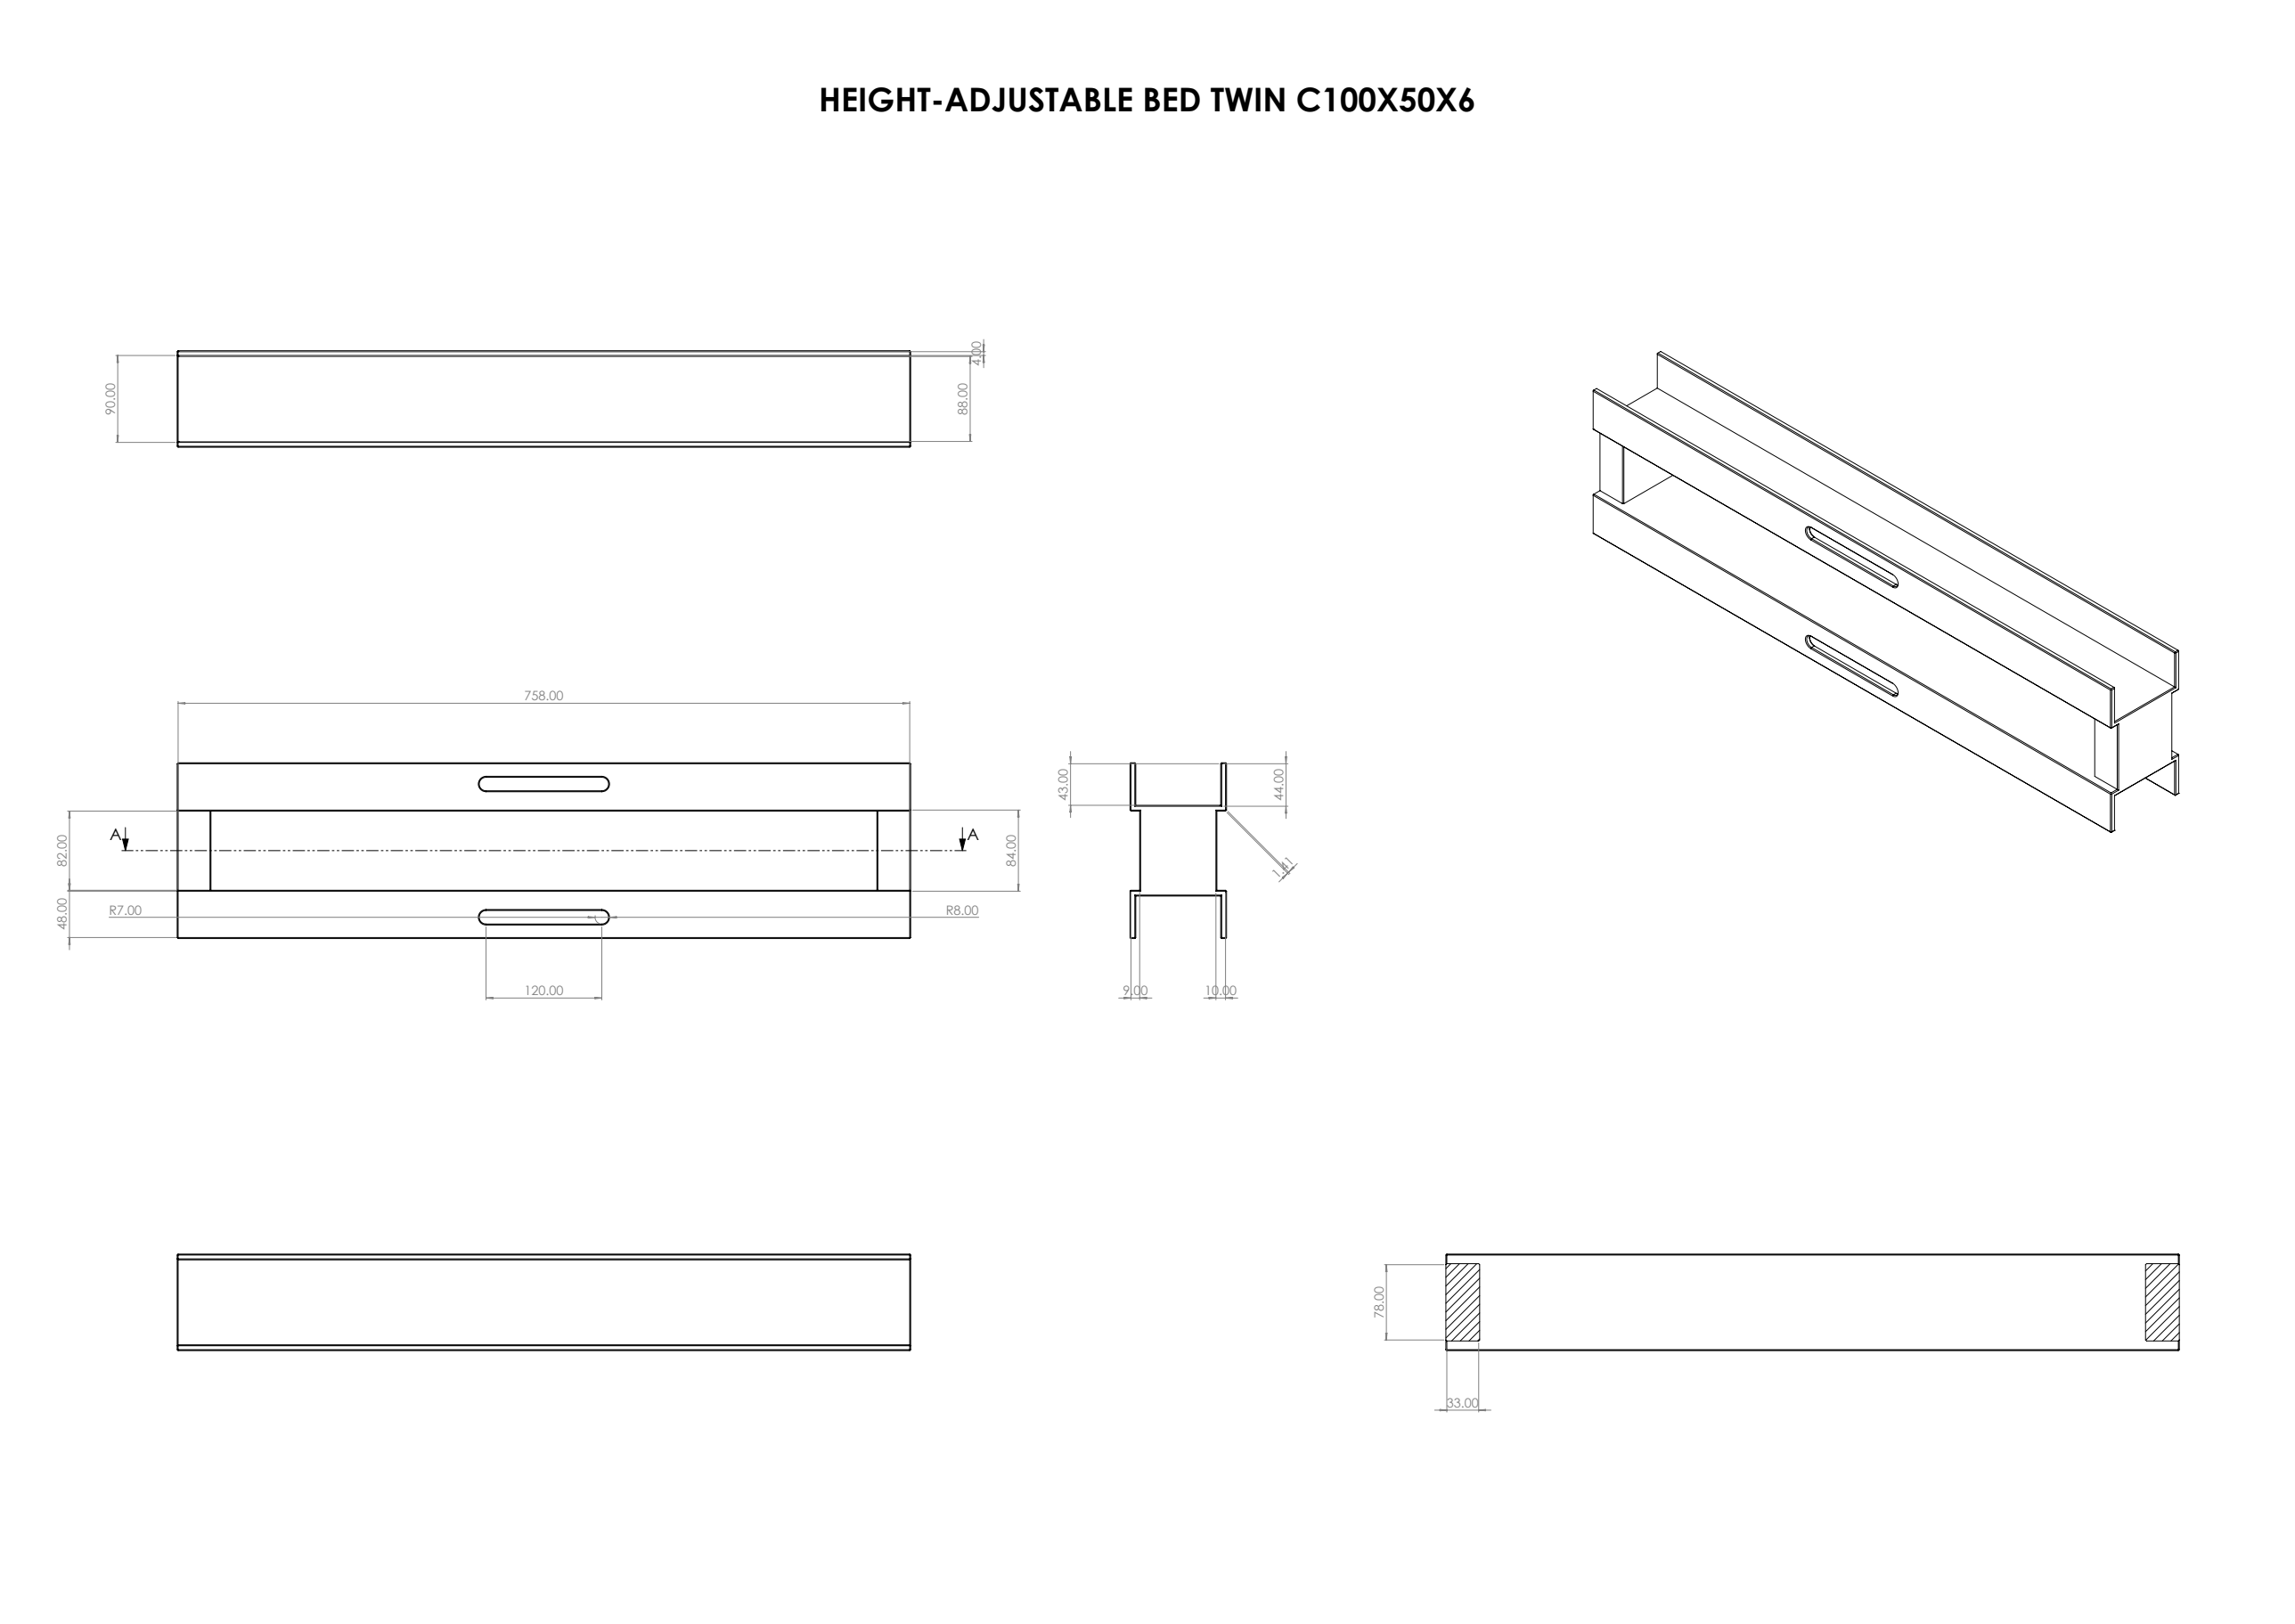
ISO-10303-21;
HEADER;
/* Generated by software containing ST-Developer
 * from STEP Tools, Inc. (www.steptools.com) 
 */

FILE_DESCRIPTION(
/* description */ (''),
/* implementation_level */ '2;1');

FILE_NAME(
/* name */ '04_Height-Adjustable_Bed_Twin_C100x50x6.step',
/* time_stamp */ '2026-10-20T10:03:03-07:00',
/* author */ (''),
/* organization */ (''),
/* preprocessor_version */ 'ST-DEVELOPER v20.2',
/* originating_system */ 'Autodesk Translation Framework v15.15.0.0',
/* authorisation */ '');

FILE_SCHEMA (('AUTOMOTIVE_DESIGN { 1 0 10303 214 3 1 1 }'));
ENDSEC;

DATA;
#10=MECHANICAL_DESIGN_GEOMETRIC_PRESENTATION_REPRESENTATION('',(#526),#71492);
#384=SHAPE_REPRESENTATION_RELATIONSHIP('SRR','None',#71605,#403);
#403=ADVANCED_BREP_SHAPE_REPRESENTATION('',(#422),#71475);
#422=MANIFOLD_SOLID_BREP('Bed',#28461);
#526=STYLED_ITEM('',(#71901),#422);
#1569=CYLINDRICAL_SURFACE('',#29276,0.7);
#1570=CYLINDRICAL_SURFACE('',#29284,0.699999999999999);
#1571=CYLINDRICAL_SURFACE('',#29291,0.699999999999999);
#1572=CYLINDRICAL_SURFACE('',#29299,0.7);
#1910=FACE_BOUND('',#5064,.T.);
#1911=FACE_BOUND('',#5070,.T.);
#1912=FACE_BOUND('',#5091,.T.);
#1913=FACE_BOUND('',#5097,.T.);
#2214=CIRCLE('',#29232,0.799999999999999);
#2215=CIRCLE('',#29233,0.8);
#2216=CIRCLE('',#29239,0.8);
#2217=CIRCLE('',#29240,0.799999999999999);
#2218=CIRCLE('',#29261,0.799999999999999);
#2219=CIRCLE('',#29262,0.8);
#2220=CIRCLE('',#29268,0.8);
#2221=CIRCLE('',#29269,0.799999999999999);
#2222=CIRCLE('',#29272,0.7);
#2223=CIRCLE('',#29275,0.699999999999999);
#2224=CIRCLE('',#29277,0.7);
#2225=CIRCLE('',#29281,0.699999999999999);
#2226=CIRCLE('',#29287,0.699999999999999);
#2227=CIRCLE('',#29290,0.7);
#2228=CIRCLE('',#29292,0.699999999999999);
#2229=CIRCLE('',#29296,0.7);
#2807=CONICAL_SURFACE('',#29271,0.75,0.785398163397475);
#2808=CONICAL_SURFACE('',#29274,0.749999999999999,0.785398163397475);
#2809=CONICAL_SURFACE('',#29280,0.749999999999999,0.785398163397475);
#2810=CONICAL_SURFACE('',#29283,0.75,0.785398163397475);
#2811=CONICAL_SURFACE('',#29286,0.749999999999999,0.785398163397475);
#2812=CONICAL_SURFACE('',#29289,0.75,0.785398163397475);
#2813=CONICAL_SURFACE('',#29295,0.75,0.785398163397475);
#2814=CONICAL_SURFACE('',#29298,0.749999999999999,0.785398163397475);
#3398=FACE_OUTER_BOUND('',#5014,.T.);
#3399=FACE_OUTER_BOUND('',#5015,.T.);
#3400=FACE_OUTER_BOUND('',#5016,.T.);
#3401=FACE_OUTER_BOUND('',#5017,.T.);
#3402=FACE_OUTER_BOUND('',#5018,.T.);
#3403=FACE_OUTER_BOUND('',#5019,.T.);
#3404=FACE_OUTER_BOUND('',#5020,.T.);
#3405=FACE_OUTER_BOUND('',#5021,.T.);
#3406=FACE_OUTER_BOUND('',#5022,.T.);
#3407=FACE_OUTER_BOUND('',#5023,.T.);
#3408=FACE_OUTER_BOUND('',#5024,.T.);
#3409=FACE_OUTER_BOUND('',#5025,.T.);
#3410=FACE_OUTER_BOUND('',#5026,.T.);
#3411=FACE_OUTER_BOUND('',#5027,.T.);
#3412=FACE_OUTER_BOUND('',#5028,.T.);
#3413=FACE_OUTER_BOUND('',#5029,.T.);
#3414=FACE_OUTER_BOUND('',#5030,.T.);
#3415=FACE_OUTER_BOUND('',#5031,.T.);
#3416=FACE_OUTER_BOUND('',#5032,.T.);
#3417=FACE_OUTER_BOUND('',#5033,.T.);
#3418=FACE_OUTER_BOUND('',#5034,.T.);
#3419=FACE_OUTER_BOUND('',#5035,.T.);
#3420=FACE_OUTER_BOUND('',#5036,.T.);
#3421=FACE_OUTER_BOUND('',#5037,.T.);
#3422=FACE_OUTER_BOUND('',#5038,.T.);
#3423=FACE_OUTER_BOUND('',#5039,.T.);
#3424=FACE_OUTER_BOUND('',#5040,.T.);
#3425=FACE_OUTER_BOUND('',#5041,.T.);
#3426=FACE_OUTER_BOUND('',#5042,.T.);
#3427=FACE_OUTER_BOUND('',#5043,.T.);
#3428=FACE_OUTER_BOUND('',#5044,.T.);
#3429=FACE_OUTER_BOUND('',#5045,.T.);
#3430=FACE_OUTER_BOUND('',#5046,.T.);
#3431=FACE_OUTER_BOUND('',#5047,.T.);
#3432=FACE_OUTER_BOUND('',#5048,.T.);
#3433=FACE_OUTER_BOUND('',#5049,.T.);
#3434=FACE_OUTER_BOUND('',#5050,.T.);
#3435=FACE_OUTER_BOUND('',#5051,.T.);
#3436=FACE_OUTER_BOUND('',#5052,.T.);
#3437=FACE_OUTER_BOUND('',#5053,.T.);
#3438=FACE_OUTER_BOUND('',#5054,.T.);
#3439=FACE_OUTER_BOUND('',#5055,.T.);
#3440=FACE_OUTER_BOUND('',#5056,.T.);
#3441=FACE_OUTER_BOUND('',#5057,.T.);
#3442=FACE_OUTER_BOUND('',#5058,.T.);
#3443=FACE_OUTER_BOUND('',#5059,.T.);
#3444=FACE_OUTER_BOUND('',#5060,.T.);
#3445=FACE_OUTER_BOUND('',#5061,.T.);
#3446=FACE_OUTER_BOUND('',#5062,.T.);
#3447=FACE_OUTER_BOUND('',#5063,.T.);
#3448=FACE_OUTER_BOUND('',#5065,.T.);
#3449=FACE_OUTER_BOUND('',#5066,.T.);
#3450=FACE_OUTER_BOUND('',#5067,.T.);
#3451=FACE_OUTER_BOUND('',#5068,.T.);
#3452=FACE_OUTER_BOUND('',#5069,.T.);
#3453=FACE_OUTER_BOUND('',#5071,.T.);
#3454=FACE_OUTER_BOUND('',#5072,.T.);
#3455=FACE_OUTER_BOUND('',#5073,.T.);
#3456=FACE_OUTER_BOUND('',#5074,.T.);
#3457=FACE_OUTER_BOUND('',#5075,.T.);
#3458=FACE_OUTER_BOUND('',#5076,.T.);
#3459=FACE_OUTER_BOUND('',#5077,.T.);
#3460=FACE_OUTER_BOUND('',#5078,.T.);
#3461=FACE_OUTER_BOUND('',#5079,.T.);
#3462=FACE_OUTER_BOUND('',#5080,.T.);
#3463=FACE_OUTER_BOUND('',#5081,.T.);
#3464=FACE_OUTER_BOUND('',#5082,.T.);
#3465=FACE_OUTER_BOUND('',#5083,.T.);
#3466=FACE_OUTER_BOUND('',#5084,.T.);
#3467=FACE_OUTER_BOUND('',#5085,.T.);
#3468=FACE_OUTER_BOUND('',#5086,.T.);
#3469=FACE_OUTER_BOUND('',#5087,.T.);
#3470=FACE_OUTER_BOUND('',#5088,.T.);
#3471=FACE_OUTER_BOUND('',#5089,.T.);
#3472=FACE_OUTER_BOUND('',#5090,.T.);
#3473=FACE_OUTER_BOUND('',#5092,.T.);
#3474=FACE_OUTER_BOUND('',#5093,.T.);
#3475=FACE_OUTER_BOUND('',#5094,.T.);
#3476=FACE_OUTER_BOUND('',#5095,.T.);
#3477=FACE_OUTER_BOUND('',#5096,.T.);
#3478=FACE_OUTER_BOUND('',#5098,.T.);
#3479=FACE_OUTER_BOUND('',#5099,.T.);
#3480=FACE_OUTER_BOUND('',#5100,.T.);
#3481=FACE_OUTER_BOUND('',#5101,.T.);
#3482=FACE_OUTER_BOUND('',#5102,.T.);
#3483=FACE_OUTER_BOUND('',#5103,.T.);
#3484=FACE_OUTER_BOUND('',#5104,.T.);
#3485=FACE_OUTER_BOUND('',#5105,.T.);
#3486=FACE_OUTER_BOUND('',#5106,.T.);
#3487=FACE_OUTER_BOUND('',#5107,.T.);
#3488=FACE_OUTER_BOUND('',#5108,.T.);
#3489=FACE_OUTER_BOUND('',#5109,.T.);
#3490=FACE_OUTER_BOUND('',#5110,.T.);
#3491=FACE_OUTER_BOUND('',#5111,.T.);
#3492=FACE_OUTER_BOUND('',#5112,.T.);
#3493=FACE_OUTER_BOUND('',#5113,.T.);
#3494=FACE_OUTER_BOUND('',#5114,.T.);
#3495=FACE_OUTER_BOUND('',#5115,.T.);
#3496=FACE_OUTER_BOUND('',#5116,.T.);
#3497=FACE_OUTER_BOUND('',#5117,.T.);
#3498=FACE_OUTER_BOUND('',#5118,.T.);
#3499=FACE_OUTER_BOUND('',#5119,.T.);
#3500=FACE_OUTER_BOUND('',#5120,.T.);
#3501=FACE_OUTER_BOUND('',#5121,.T.);
#3502=FACE_OUTER_BOUND('',#5122,.T.);
#3503=FACE_OUTER_BOUND('',#5123,.T.);
#3504=FACE_OUTER_BOUND('',#5124,.T.);
#3505=FACE_OUTER_BOUND('',#5125,.T.);
#5014=EDGE_LOOP('',(#20251,#20252,#20253,#20254));
#5015=EDGE_LOOP('',(#20255,#20256,#20257,#20258));
#5016=EDGE_LOOP('',(#20259,#20260,#20261,#20262,#20263,#20264));
#5017=EDGE_LOOP('',(#20265,#20266,#20267,#20268));
#5018=EDGE_LOOP('',(#20269,#20270,#20271,#20272,#20273,#20274));
#5019=EDGE_LOOP('',(#20275,#20276,#20277,#20278,#20279,#20280));
#5020=EDGE_LOOP('',(#20281,#20282,#20283,#20284));
#5021=EDGE_LOOP('',(#20285,#20286,#20287,#20288));
#5022=EDGE_LOOP('',(#20289,#20290,#20291,#20292));
#5023=EDGE_LOOP('',(#20293,#20294,#20295,#20296));
#5024=EDGE_LOOP('',(#20297,#20298,#20299,#20300,#20301,#20302));
#5025=EDGE_LOOP('',(#20303,#20304,#20305,#20306,#20307,#20308));
#5026=EDGE_LOOP('',(#20309,#20310,#20311,#20312));
#5027=EDGE_LOOP('',(#20313,#20314,#20315,#20316,#20317,#20318));
#5028=EDGE_LOOP('',(#20319,#20320,#20321,#20322,#20323,#20324));
#5029=EDGE_LOOP('',(#20325,#20326,#20327,#20328,#20329));
#5030=EDGE_LOOP('',(#20330,#20331,#20332,#20333));
#5031=EDGE_LOOP('',(#20334,#20335,#20336,#20337,#20338,#20339));
#5032=EDGE_LOOP('',(#20340,#20341,#20342,#20343,#20344));
#5033=EDGE_LOOP('',(#20345,#20346,#20347,#20348));
#5034=EDGE_LOOP('',(#20349,#20350,#20351,#20352));
#5035=EDGE_LOOP('',(#20353,#20354,#20355,#20356));
#5036=EDGE_LOOP('',(#20357,#20358,#20359,#20360));
#5037=EDGE_LOOP('',(#20361,#20362,#20363,#20364));
#5038=EDGE_LOOP('',(#20365,#20366,#20367));
#5039=EDGE_LOOP('',(#20368,#20369,#20370,#20371,#20372));
#5040=EDGE_LOOP('',(#20373,#20374,#20375));
#5041=EDGE_LOOP('',(#20376,#20377,#20378,#20379,#20380));
#5042=EDGE_LOOP('',(#20381,#20382,#20383,#20384,#20385));
#5043=EDGE_LOOP('',(#20386,#20387,#20388,#20389));
#5044=EDGE_LOOP('',(#20390,#20391,#20392,#20393));
#5045=EDGE_LOOP('',(#20394,#20395,#20396,#20397));
#5046=EDGE_LOOP('',(#20398,#20399,#20400,#20401,#20402));
#5047=EDGE_LOOP('',(#20403,#20404,#20405,#20406,#20407,#20408,#20409,#20410,
#20411,#20412,#20413,#20414,#20415,#20416,#20417,#20418,#20419,#20420,#20421,
#20422));
#5048=EDGE_LOOP('',(#20423,#20424,#20425,#20426,#20427,#20428));
#5049=EDGE_LOOP('',(#20429,#20430,#20431,#20432,#20433));
#5050=EDGE_LOOP('',(#20434,#20435,#20436,#20437));
#5051=EDGE_LOOP('',(#20438,#20439,#20440,#20441,#20442));
#5052=EDGE_LOOP('',(#20443,#20444,#20445,#20446));
#5053=EDGE_LOOP('',(#20447,#20448,#20449,#20450,#20451));
#5054=EDGE_LOOP('',(#20452,#20453,#20454,#20455));
#5055=EDGE_LOOP('',(#20456,#20457,#20458));
#5056=EDGE_LOOP('',(#20459,#20460,#20461,#20462,#20463));
#5057=EDGE_LOOP('',(#20464,#20465,#20466,#20467));
#5058=EDGE_LOOP('',(#20468,#20469,#20470,#20471,#20472));
#5059=EDGE_LOOP('',(#20473,#20474,#20475,#20476));
#5060=EDGE_LOOP('',(#20477,#20478,#20479,#20480,#20481,#20482,#20483,#20484,
#20485,#20486,#20487,#20488,#20489,#20490,#20491,#20492));
#5061=EDGE_LOOP('',(#20493,#20494,#20495,#20496,#20497));
#5062=EDGE_LOOP('',(#20498,#20499,#20500,#20501,#20502,#20503));
#5063=EDGE_LOOP('',(#20504,#20505,#20506,#20507));
#5064=EDGE_LOOP('',(#20508,#20509,#20510,#20511));
#5065=EDGE_LOOP('',(#20512,#20513,#20514,#20515,#20516,#20517));
#5066=EDGE_LOOP('',(#20518,#20519,#20520,#20521,#20522,#20523));
#5067=EDGE_LOOP('',(#20524,#20525,#20526,#20527,#20528,#20529));
#5068=EDGE_LOOP('',(#20530,#20531,#20532,#20533,#20534));
#5069=EDGE_LOOP('',(#20535,#20536,#20537,#20538));
#5070=EDGE_LOOP('',(#20539,#20540,#20541,#20542));
#5071=EDGE_LOOP('',(#20543,#20544,#20545,#20546,#20547));
#5072=EDGE_LOOP('',(#20548,#20549,#20550,#20551,#20552,#20553));
#5073=EDGE_LOOP('',(#20554,#20555,#20556,#20557));
#5074=EDGE_LOOP('',(#20558,#20559,#20560,#20561,#20562));
#5075=EDGE_LOOP('',(#20563,#20564,#20565,#20566,#20567,#20568,#20569,#20570,
#20571,#20572,#20573,#20574,#20575,#20576,#20577,#20578,#20579,#20580,#20581,
#20582));
#5076=EDGE_LOOP('',(#20583,#20584,#20585,#20586));
#5077=EDGE_LOOP('',(#20587,#20588,#20589,#20590));
#5078=EDGE_LOOP('',(#20591,#20592,#20593));
#5079=EDGE_LOOP('',(#20594,#20595,#20596,#20597));
#5080=EDGE_LOOP('',(#20598,#20599,#20600,#20601,#20602));
#5081=EDGE_LOOP('',(#20603,#20604,#20605,#20606,#20607));
#5082=EDGE_LOOP('',(#20608,#20609,#20610,#20611));
#5083=EDGE_LOOP('',(#20612,#20613,#20614,#20615,#20616,#20617));
#5084=EDGE_LOOP('',(#20618,#20619,#20620,#20621));
#5085=EDGE_LOOP('',(#20622,#20623,#20624,#20625,#20626,#20627,#20628,#20629,
#20630,#20631,#20632,#20633,#20634,#20635,#20636,#20637));
#5086=EDGE_LOOP('',(#20638,#20639,#20640,#20641,#20642,#20643));
#5087=EDGE_LOOP('',(#20644,#20645,#20646,#20647));
#5088=EDGE_LOOP('',(#20648,#20649,#20650,#20651,#20652));
#5089=EDGE_LOOP('',(#20653,#20654,#20655,#20656,#20657));
#5090=EDGE_LOOP('',(#20658,#20659,#20660,#20661));
#5091=EDGE_LOOP('',(#20662,#20663,#20664,#20665));
#5092=EDGE_LOOP('',(#20666,#20667,#20668,#20669,#20670,#20671));
#5093=EDGE_LOOP('',(#20672,#20673,#20674,#20675,#20676));
#5094=EDGE_LOOP('',(#20677,#20678,#20679,#20680,#20681,#20682));
#5095=EDGE_LOOP('',(#20683,#20684,#20685,#20686,#20687,#20688));
#5096=EDGE_LOOP('',(#20689,#20690,#20691,#20692));
#5097=EDGE_LOOP('',(#20693,#20694,#20695,#20696));
#5098=EDGE_LOOP('',(#20697,#20698,#20699,#20700));
#5099=EDGE_LOOP('',(#20701,#20702,#20703,#20704));
#5100=EDGE_LOOP('',(#20705,#20706,#20707,#20708));
#5101=EDGE_LOOP('',(#20709,#20710,#20711,#20712));
#5102=EDGE_LOOP('',(#20713,#20714,#20715,#20716));
#5103=EDGE_LOOP('',(#20717,#20718,#20719,#20720));
#5104=EDGE_LOOP('',(#20721,#20722,#20723,#20724));
#5105=EDGE_LOOP('',(#20725,#20726,#20727,#20728));
#5106=EDGE_LOOP('',(#20729,#20730,#20731,#20732));
#5107=EDGE_LOOP('',(#20733,#20734,#20735,#20736));
#5108=EDGE_LOOP('',(#20737,#20738,#20739,#20740));
#5109=EDGE_LOOP('',(#20741,#20742,#20743,#20744));
#5110=EDGE_LOOP('',(#20745,#20746,#20747,#20748));
#5111=EDGE_LOOP('',(#20749,#20750,#20751,#20752));
#5112=EDGE_LOOP('',(#20753,#20754,#20755,#20756));
#5113=EDGE_LOOP('',(#20757,#20758,#20759,#20760));
#5114=EDGE_LOOP('',(#20761,#20762,#20763,#20764));
#5115=EDGE_LOOP('',(#20765,#20766,#20767,#20768));
#5116=EDGE_LOOP('',(#20769,#20770,#20771,#20772));
#5117=EDGE_LOOP('',(#20773,#20774,#20775,#20776));
#5118=EDGE_LOOP('',(#20777,#20778,#20779,#20780));
#5119=EDGE_LOOP('',(#20781,#20782,#20783,#20784));
#5120=EDGE_LOOP('',(#20785,#20786,#20787,#20788));
#5121=EDGE_LOOP('',(#20789,#20790,#20791,#20792));
#5122=EDGE_LOOP('',(#20793,#20794,#20795,#20796));
#5123=EDGE_LOOP('',(#20797,#20798,#20799,#20800,#20801,#20802));
#5124=EDGE_LOOP('',(#20803,#20804,#20805,#20806));
#5125=EDGE_LOOP('',(#20807,#20808,#20809,#20810));
#7065=LINE('',#42807,#9553);
#7066=LINE('',#42809,#9554);
#7067=LINE('',#42811,#9555);
#7068=LINE('',#42812,#9556);
#7069=LINE('',#42815,#9557);
#7070=LINE('',#42817,#9558);
#7071=LINE('',#42818,#9559);
#7072=LINE('',#42822,#9560);
#7073=LINE('',#42824,#9561);
#7074=LINE('',#42826,#9562);
#7075=LINE('',#42828,#9563);
#7076=LINE('',#42830,#9564);
#7077=LINE('',#42831,#9565);
#7078=LINE('',#42834,#9566);
#7079=LINE('',#42836,#9567);
#7080=LINE('',#42837,#9568);
#7081=LINE('',#42840,#9569);
#7082=LINE('',#42842,#9570);
#7083=LINE('',#42844,#9571);
#7084=LINE('',#42845,#9572);
#7085=LINE('',#42848,#9573);
#7086=LINE('',#42850,#9574);
#7087=LINE('',#42852,#9575);
#7088=LINE('',#42853,#9576);
#7089=LINE('',#42857,#9577);
#7090=LINE('',#42859,#9578);
#7091=LINE('',#42861,#9579);
#7092=LINE('',#42862,#9580);
#7093=LINE('',#42864,#9581);
#7094=LINE('',#42865,#9582);
#7095=LINE('',#42869,#9583);
#7096=LINE('',#42871,#9584);
#7097=LINE('',#42873,#9585);
#7098=LINE('',#42874,#9586);
#7099=LINE('',#42877,#9587);
#7100=LINE('',#42879,#9588);
#7101=LINE('',#42880,#9589);
#7102=LINE('',#42884,#9590);
#7103=LINE('',#42886,#9591);
#7104=LINE('',#42888,#9592);
#7105=LINE('',#42890,#9593);
#7106=LINE('',#42892,#9594);
#7107=LINE('',#42893,#9595);
#7108=LINE('',#42896,#9596);
#7109=LINE('',#42898,#9597);
#7110=LINE('',#42900,#9598);
#7111=LINE('',#42902,#9599);
#7112=LINE('',#42903,#9600);
#7113=LINE('',#42906,#9601);
#7114=LINE('',#42907,#9602);
#7115=LINE('',#42910,#9603);
#7116=LINE('',#42912,#9604);
#7117=LINE('',#42914,#9605);
#7118=LINE('',#42915,#9606);
#7119=LINE('',#42918,#9607);
#7120=LINE('',#42920,#9608);
#7121=LINE('',#42921,#9609);
#7122=LINE('',#42924,#9610);
#7123=LINE('',#42926,#9611);
#7124=LINE('',#42927,#9612);
#7125=LINE('',#42930,#9613);
#7126=LINE('',#42931,#9614);
#7127=LINE('',#42934,#9615);
#7128=LINE('',#42936,#9616);
#7129=LINE('',#42937,#9617);
#7130=LINE('',#42940,#9618);
#7131=LINE('',#42942,#9619);
#7132=LINE('',#42943,#9620);
#7133=LINE('',#42946,#9621);
#7134=LINE('',#42948,#9622);
#7135=LINE('',#42949,#9623);
#7136=LINE('',#42952,#9624);
#7137=LINE('',#42953,#9625);
#7138=LINE('',#42956,#9626);
#7139=LINE('',#42957,#9627);
#7140=LINE('',#42961,#9628);
#7141=LINE('',#42963,#9629);
#7142=LINE('',#42965,#9630);
#7143=LINE('',#42966,#9631);
#7144=LINE('',#42968,#9632);
#7145=LINE('',#42969,#9633);
#7146=LINE('',#42972,#9634);
#7147=LINE('',#42973,#9635);
#7148=LINE('',#42976,#9636);
#7149=LINE('',#42977,#9637);
#7150=LINE('',#42981,#9638);
#7151=LINE('',#42983,#9639);
#7152=LINE('',#42984,#9640);
#7153=LINE('',#42986,#9641);
#7154=LINE('',#42988,#9642);
#7155=LINE('',#42989,#9643);
#7156=LINE('',#42992,#9644);
#7157=LINE('',#42993,#9645);
#7158=LINE('',#42994,#9646);
#7159=LINE('',#42996,#9647);
#7160=LINE('',#42998,#9648);
#7161=LINE('',#42999,#9649);
#7162=LINE('',#43002,#9650);
#7163=LINE('',#43003,#9651);
#7164=LINE('',#43005,#9652);
#7165=LINE('',#43006,#9653);
#7166=LINE('',#43009,#9654);
#7167=LINE('',#43010,#9655);
#7168=LINE('',#43011,#9656);
#7169=LINE('',#43014,#9657);
#7170=LINE('',#43016,#9658);
#7171=LINE('',#43018,#9659);
#7172=LINE('',#43020,#9660);
#7173=LINE('',#43022,#9661);
#7174=LINE('',#43024,#9662);
#7175=LINE('',#43026,#9663);
#7176=LINE('',#43028,#9664);
#7177=LINE('',#43030,#9665);
#7178=LINE('',#43032,#9666);
#7179=LINE('',#43034,#9667);
#7180=LINE('',#43035,#9668);
#7181=LINE('',#43038,#9669);
#7182=LINE('',#43040,#9670);
#7183=LINE('',#43042,#9671);
#7184=LINE('',#43043,#9672);
#7185=LINE('',#43046,#9673);
#7186=LINE('',#43047,#9674);
#7187=LINE('',#43048,#9675);
#7188=LINE('',#43051,#9676);
#7189=LINE('',#43052,#9677);
#7190=LINE('',#43055,#9678);
#7191=LINE('',#43056,#9679);
#7192=LINE('',#43059,#9680);
#7193=LINE('',#43060,#9681);
#7194=LINE('',#43064,#9682);
#7195=LINE('',#43066,#9683);
#7196=LINE('',#43067,#9684);
#7197=LINE('',#43068,#9685);
#7198=LINE('',#43071,#9686);
#7199=LINE('',#43072,#9687);
#7200=LINE('',#43075,#9688);
#7201=LINE('',#43077,#9689);
#7202=LINE('',#43078,#9690);
#7203=LINE('',#43082,#9691);
#7204=LINE('',#43083,#9692);
#7205=LINE('',#43085,#9693);
#7206=LINE('',#43086,#9694);
#7207=LINE('',#43088,#9695);
#7208=LINE('',#43092,#9696);
#7209=LINE('',#43093,#9697);
#7210=LINE('',#43094,#9698);
#7211=LINE('',#43096,#9699);
#7212=LINE('',#43097,#9700);
#7213=LINE('',#43100,#9701);
#7214=LINE('',#43101,#9702);
#7215=LINE('',#43102,#9703);
#7216=LINE('',#43105,#9704);
#7217=LINE('',#43107,#9705);
#7218=LINE('',#43108,#9706);
#7219=LINE('',#43111,#9707);
#7220=LINE('',#43113,#9708);
#7221=LINE('',#43115,#9709);
#7222=LINE('',#43116,#9710);
#7223=LINE('',#43118,#9711);
#7224=LINE('',#43121,#9712);
#7225=LINE('',#43125,#9713);
#7226=LINE('',#43129,#9714);
#7227=LINE('',#43131,#9715);
#7228=LINE('',#43132,#9716);
#7229=LINE('',#43135,#9717);
#7230=LINE('',#43137,#9718);
#7231=LINE('',#43139,#9719);
#7232=LINE('',#43140,#9720);
#7233=LINE('',#43144,#9721);
#7234=LINE('',#43146,#9722);
#7235=LINE('',#43147,#9723);
#7236=LINE('',#43149,#9724);
#7237=LINE('',#43150,#9725);
#7238=LINE('',#43153,#9726);
#7239=LINE('',#43155,#9727);
#7240=LINE('',#43156,#9728);
#7241=LINE('',#43158,#9729);
#7242=LINE('',#43159,#9730);
#7243=LINE('',#43162,#9731);
#7244=LINE('',#43166,#9732);
#7245=LINE('',#43169,#9733);
#7246=LINE('',#43171,#9734);
#7247=LINE('',#43174,#9735);
#7248=LINE('',#43175,#9736);
#7249=LINE('',#43177,#9737);
#7250=LINE('',#43180,#9738);
#7251=LINE('',#43182,#9739);
#7252=LINE('',#43184,#9740);
#7253=LINE('',#43186,#9741);
#7254=LINE('',#43188,#9742);
#7255=LINE('',#43190,#9743);
#7256=LINE('',#43191,#9744);
#7257=LINE('',#43192,#9745);
#7258=LINE('',#43194,#9746);
#7259=LINE('',#43199,#9747);
#7260=LINE('',#43200,#9748);
#7261=LINE('',#43201,#9749);
#7262=LINE('',#43204,#9750);
#7263=LINE('',#43205,#9751);
#7264=LINE('',#43209,#9752);
#7265=LINE('',#43210,#9753);
#7266=LINE('',#43211,#9754);
#7267=LINE('',#43213,#9755);
#7268=LINE('',#43215,#9756);
#7269=LINE('',#43216,#9757);
#7270=LINE('',#43218,#9758);
#7271=LINE('',#43221,#9759);
#7272=LINE('',#43223,#9760);
#7273=LINE('',#43224,#9761);
#7274=LINE('',#43226,#9762);
#7275=LINE('',#43230,#9763);
#7276=LINE('',#43232,#9764);
#7277=LINE('',#43234,#9765);
#7278=LINE('',#43235,#9766);
#7279=LINE('',#43237,#9767);
#7280=LINE('',#43238,#9768);
#7281=LINE('',#43242,#9769);
#7282=LINE('',#43243,#9770);
#7283=LINE('',#43246,#9771);
#7284=LINE('',#43247,#9772);
#7285=LINE('',#43250,#9773);
#7286=LINE('',#43254,#9774);
#7287=LINE('',#43258,#9775);
#7288=LINE('',#43260,#9776);
#7289=LINE('',#43261,#9777);
#7290=LINE('',#43263,#9778);
#7291=LINE('',#43266,#9779);
#7292=LINE('',#43267,#9780);
#7293=LINE('',#43269,#9781);
#7294=LINE('',#43270,#9782);
#7295=LINE('',#43274,#9783);
#7296=LINE('',#43278,#9784);
#7297=LINE('',#43282,#9785);
#7298=LINE('',#43284,#9786);
#7299=LINE('',#43285,#9787);
#7300=LINE('',#43288,#9788);
#7301=LINE('',#43292,#9789);
#7302=LINE('',#43293,#9790);
#7303=LINE('',#43298,#9791);
#7304=LINE('',#43301,#9792);
#7305=LINE('',#43304,#9793);
#7306=LINE('',#43305,#9794);
#7307=LINE('',#43307,#9795);
#7308=LINE('',#43308,#9796);
#7309=LINE('',#43311,#9797);
#7310=LINE('',#43314,#9798);
#7311=LINE('',#43315,#9799);
#7312=LINE('',#43318,#9800);
#7313=LINE('',#43321,#9801);
#7314=LINE('',#43323,#9802);
#7315=LINE('',#43324,#9803);
#7316=LINE('',#43327,#9804);
#7317=LINE('',#43331,#9805);
#7318=LINE('',#43332,#9806);
#7319=LINE('',#43337,#9807);
#7320=LINE('',#43340,#9808);
#7321=LINE('',#43343,#9809);
#7322=LINE('',#43344,#9810);
#7323=LINE('',#43346,#9811);
#7324=LINE('',#43347,#9812);
#7325=LINE('',#43350,#9813);
#7326=LINE('',#43353,#9814);
#7327=LINE('',#43354,#9815);
#7328=LINE('',#43357,#9816);
#9553=VECTOR('',#32608,1.);
#9554=VECTOR('',#32609,1.);
#9555=VECTOR('',#32610,1.);
#9556=VECTOR('',#32611,1.);
#9557=VECTOR('',#32614,1.);
#9558=VECTOR('',#32615,1.);
#9559=VECTOR('',#32616,1.);
#9560=VECTOR('',#32619,1.);
#9561=VECTOR('',#32620,1.);
#9562=VECTOR('',#32621,1.);
#9563=VECTOR('',#32622,1.);
#9564=VECTOR('',#32623,1.);
#9565=VECTOR('',#32624,1.);
#9566=VECTOR('',#32627,1.);
#9567=VECTOR('',#32628,1.);
#9568=VECTOR('',#32629,1.);
#9569=VECTOR('',#32632,1.);
#9570=VECTOR('',#32633,1.);
#9571=VECTOR('',#32634,1.);
#9572=VECTOR('',#32635,1.);
#9573=VECTOR('',#32638,1.);
#9574=VECTOR('',#32639,1.);
#9575=VECTOR('',#32640,1.);
#9576=VECTOR('',#32641,1.);
#9577=VECTOR('',#32644,1.);
#9578=VECTOR('',#32645,1.);
#9579=VECTOR('',#32646,1.);
#9580=VECTOR('',#32647,1.);
#9581=VECTOR('',#32650,1.);
#9582=VECTOR('',#32651,1.);
#9583=VECTOR('',#32654,1.);
#9584=VECTOR('',#32655,1.);
#9585=VECTOR('',#32656,1.);
#9586=VECTOR('',#32657,1.);
#9587=VECTOR('',#32660,1.);
#9588=VECTOR('',#32661,1.);
#9589=VECTOR('',#32662,1.);
#9590=VECTOR('',#32665,1.);
#9591=VECTOR('',#32666,1.);
#9592=VECTOR('',#32667,1.);
#9593=VECTOR('',#32668,1.);
#9594=VECTOR('',#32669,1.);
#9595=VECTOR('',#32670,1.);
#9596=VECTOR('',#32673,1.);
#9597=VECTOR('',#32674,1.);
#9598=VECTOR('',#32675,1.);
#9599=VECTOR('',#32676,1.);
#9600=VECTOR('',#32677,1.);
#9601=VECTOR('',#32680,1.);
#9602=VECTOR('',#32681,1.);
#9603=VECTOR('',#32684,1.);
#9604=VECTOR('',#32685,1.);
#9605=VECTOR('',#32686,1.);
#9606=VECTOR('',#32687,1.);
#9607=VECTOR('',#32690,1.);
#9608=VECTOR('',#32691,1.);
#9609=VECTOR('',#32692,1.);
#9610=VECTOR('',#32695,1.);
#9611=VECTOR('',#32696,1.);
#9612=VECTOR('',#32697,1.);
#9613=VECTOR('',#32700,1.);
#9614=VECTOR('',#32701,1.);
#9615=VECTOR('',#32704,1.);
#9616=VECTOR('',#32705,1.);
#9617=VECTOR('',#32706,1.);
#9618=VECTOR('',#32709,1.);
#9619=VECTOR('',#32710,1.);
#9620=VECTOR('',#32711,1.);
#9621=VECTOR('',#32714,1.);
#9622=VECTOR('',#32715,1.);
#9623=VECTOR('',#32716,1.);
#9624=VECTOR('',#32719,1.);
#9625=VECTOR('',#32720,1.);
#9626=VECTOR('',#32723,1.);
#9627=VECTOR('',#32724,1.);
#9628=VECTOR('',#32727,1.);
#9629=VECTOR('',#32728,1.);
#9630=VECTOR('',#32729,1.);
#9631=VECTOR('',#32730,1.);
#9632=VECTOR('',#32733,1.);
#9633=VECTOR('',#32734,1.);
#9634=VECTOR('',#32737,1.);
#9635=VECTOR('',#32738,1.);
#9636=VECTOR('',#32741,1.);
#9637=VECTOR('',#32742,1.);
#9638=VECTOR('',#32745,1.);
#9639=VECTOR('',#32746,1.);
#9640=VECTOR('',#32747,1.);
#9641=VECTOR('',#32750,1.);
#9642=VECTOR('',#32751,1.);
#9643=VECTOR('',#32752,1.);
#9644=VECTOR('',#32755,1.);
#9645=VECTOR('',#32756,1.);
#9646=VECTOR('',#32757,1.);
#9647=VECTOR('',#32760,1.);
#9648=VECTOR('',#32761,1.);
#9649=VECTOR('',#32762,1.);
#9650=VECTOR('',#32765,1.);
#9651=VECTOR('',#32766,1.);
#9652=VECTOR('',#32769,1.);
#9653=VECTOR('',#32770,1.);
#9654=VECTOR('',#32773,1.);
#9655=VECTOR('',#32774,1.);
#9656=VECTOR('',#32775,1.);
#9657=VECTOR('',#32778,1.);
#9658=VECTOR('',#32779,1.);
#9659=VECTOR('',#32780,1.);
#9660=VECTOR('',#32781,1.);
#9661=VECTOR('',#32782,1.);
#9662=VECTOR('',#32783,1.);
#9663=VECTOR('',#32784,1.);
#9664=VECTOR('',#32785,1.);
#9665=VECTOR('',#32786,1.);
#9666=VECTOR('',#32787,1.);
#9667=VECTOR('',#32788,1.);
#9668=VECTOR('',#32789,1.);
#9669=VECTOR('',#32792,1.);
#9670=VECTOR('',#32793,1.);
#9671=VECTOR('',#32794,1.);
#9672=VECTOR('',#32795,1.);
#9673=VECTOR('',#32798,1.);
#9674=VECTOR('',#32799,1.);
#9675=VECTOR('',#32800,1.);
#9676=VECTOR('',#32803,1.);
#9677=VECTOR('',#32804,1.);
#9678=VECTOR('',#32807,1.);
#9679=VECTOR('',#32808,1.);
#9680=VECTOR('',#32811,1.);
#9681=VECTOR('',#32812,1.);
#9682=VECTOR('',#32815,1.);
#9683=VECTOR('',#32816,1.);
#9684=VECTOR('',#32817,1.);
#9685=VECTOR('',#32818,1.);
#9686=VECTOR('',#32821,1.);
#9687=VECTOR('',#32822,1.);
#9688=VECTOR('',#32825,1.);
#9689=VECTOR('',#32826,1.);
#9690=VECTOR('',#32827,1.);
#9691=VECTOR('',#32830,1.);
#9692=VECTOR('',#32831,1.);
#9693=VECTOR('',#32832,1.);
#9694=VECTOR('',#32833,1.);
#9695=VECTOR('',#32836,1.);
#9696=VECTOR('',#32839,1.);
#9697=VECTOR('',#32840,1.);
#9698=VECTOR('',#32841,1.);
#9699=VECTOR('',#32844,1.);
#9700=VECTOR('',#32845,1.);
#9701=VECTOR('',#32848,1.);
#9702=VECTOR('',#32849,1.);
#9703=VECTOR('',#32850,1.);
#9704=VECTOR('',#32853,1.);
#9705=VECTOR('',#32854,1.);
#9706=VECTOR('',#32855,1.);
#9707=VECTOR('',#32858,1.);
#9708=VECTOR('',#32859,1.);
#9709=VECTOR('',#32860,1.);
#9710=VECTOR('',#32861,1.);
#9711=VECTOR('',#32864,1.);
#9712=VECTOR('',#32865,1.);
#9713=VECTOR('',#32868,1.);
#9714=VECTOR('',#32873,1.);
#9715=VECTOR('',#32874,1.);
#9716=VECTOR('',#32875,1.);
#9717=VECTOR('',#32878,1.);
#9718=VECTOR('',#32879,1.);
#9719=VECTOR('',#32880,1.);
#9720=VECTOR('',#32881,1.);
#9721=VECTOR('',#32884,1.);
#9722=VECTOR('',#32885,1.);
#9723=VECTOR('',#32886,1.);
#9724=VECTOR('',#32887,1.);
#9725=VECTOR('',#32888,1.);
#9726=VECTOR('',#32891,1.);
#9727=VECTOR('',#32892,1.);
#9728=VECTOR('',#32893,1.);
#9729=VECTOR('',#32896,1.);
#9730=VECTOR('',#32897,1.);
#9731=VECTOR('',#32898,1.);
#9732=VECTOR('',#32901,1.);
#9733=VECTOR('',#32906,1.);
#9734=VECTOR('',#32909,1.);
#9735=VECTOR('',#32912,1.);
#9736=VECTOR('',#32913,1.);
#9737=VECTOR('',#32916,1.);
#9738=VECTOR('',#32919,1.);
#9739=VECTOR('',#32920,1.);
#9740=VECTOR('',#32921,1.);
#9741=VECTOR('',#32922,1.);
#9742=VECTOR('',#32923,1.);
#9743=VECTOR('',#32924,1.);
#9744=VECTOR('',#32925,1.);
#9745=VECTOR('',#32926,1.);
#9746=VECTOR('',#32929,1.);
#9747=VECTOR('',#32934,1.);
#9748=VECTOR('',#32935,1.);
#9749=VECTOR('',#32936,1.);
#9750=VECTOR('',#32939,1.);
#9751=VECTOR('',#32940,1.);
#9752=VECTOR('',#32943,1.);
#9753=VECTOR('',#32944,1.);
#9754=VECTOR('',#32945,1.);
#9755=VECTOR('',#32948,1.);
#9756=VECTOR('',#32949,1.);
#9757=VECTOR('',#32950,1.);
#9758=VECTOR('',#32953,1.);
#9759=VECTOR('',#32956,1.);
#9760=VECTOR('',#32957,1.);
#9761=VECTOR('',#32958,1.);
#9762=VECTOR('',#32961,1.);
#9763=VECTOR('',#32966,1.);
#9764=VECTOR('',#32967,1.);
#9765=VECTOR('',#32968,1.);
#9766=VECTOR('',#32969,1.);
#9767=VECTOR('',#32972,1.);
#9768=VECTOR('',#32973,1.);
#9769=VECTOR('',#32978,1.);
#9770=VECTOR('',#32979,1.);
#9771=VECTOR('',#32982,1.);
#9772=VECTOR('',#32983,1.);
#9773=VECTOR('',#32984,1.);
#9774=VECTOR('',#32987,1.);
#9775=VECTOR('',#32992,1.);
#9776=VECTOR('',#32993,1.);
#9777=VECTOR('',#32994,1.);
#9778=VECTOR('',#32997,1.);
#9779=VECTOR('',#33000,1.);
#9780=VECTOR('',#33001,1.);
#9781=VECTOR('',#33004,1.);
#9782=VECTOR('',#33005,1.);
#9783=VECTOR('',#33008,1.);
#9784=VECTOR('',#33011,1.);
#9785=VECTOR('',#33016,1.);
#9786=VECTOR('',#33017,1.);
#9787=VECTOR('',#33018,1.);
#9788=VECTOR('',#33021,1.);
#9789=VECTOR('',#33026,1.);
#9790=VECTOR('',#33027,1.);
#9791=VECTOR('',#33034,1.);
#9792=VECTOR('',#33037,1.);
#9793=VECTOR('',#33040,1.);
#9794=VECTOR('',#33041,1.);
#9795=VECTOR('',#33044,1.);
#9796=VECTOR('',#33045,1.);
#9797=VECTOR('',#33048,1.);
#9798=VECTOR('',#33053,1.);
#9799=VECTOR('',#33054,1.);
#9800=VECTOR('',#33059,1.);
#9801=VECTOR('',#33062,1.);
#9802=VECTOR('',#33063,1.);
#9803=VECTOR('',#33064,1.);
#9804=VECTOR('',#33067,1.);
#9805=VECTOR('',#33072,1.);
#9806=VECTOR('',#33073,1.);
#9807=VECTOR('',#33080,1.);
#9808=VECTOR('',#33083,1.);
#9809=VECTOR('',#33086,1.);
#9810=VECTOR('',#33087,1.);
#9811=VECTOR('',#33090,1.);
#9812=VECTOR('',#33091,1.);
#9813=VECTOR('',#33094,1.);
#9814=VECTOR('',#33099,1.);
#9815=VECTOR('',#33100,1.);
#9816=VECTOR('',#33105,1.);
#12011=VERTEX_POINT('',#42805);
#12012=VERTEX_POINT('',#42806);
#12013=VERTEX_POINT('',#42808);
#12014=VERTEX_POINT('',#42810);
#12015=VERTEX_POINT('',#42814);
#12016=VERTEX_POINT('',#42816);
#12017=VERTEX_POINT('',#42820);
#12018=VERTEX_POINT('',#42821);
#12019=VERTEX_POINT('',#42823);
#12020=VERTEX_POINT('',#42825);
#12021=VERTEX_POINT('',#42827);
#12022=VERTEX_POINT('',#42829);
#12023=VERTEX_POINT('',#42833);
#12024=VERTEX_POINT('',#42835);
#12025=VERTEX_POINT('',#42839);
#12026=VERTEX_POINT('',#42841);
#12027=VERTEX_POINT('',#42843);
#12028=VERTEX_POINT('',#42847);
#12029=VERTEX_POINT('',#42849);
#12030=VERTEX_POINT('',#42851);
#12031=VERTEX_POINT('',#42855);
#12032=VERTEX_POINT('',#42856);
#12033=VERTEX_POINT('',#42858);
#12034=VERTEX_POINT('',#42860);
#12035=VERTEX_POINT('',#42867);
#12036=VERTEX_POINT('',#42868);
#12037=VERTEX_POINT('',#42870);
#12038=VERTEX_POINT('',#42872);
#12039=VERTEX_POINT('',#42876);
#12040=VERTEX_POINT('',#42878);
#12041=VERTEX_POINT('',#42882);
#12042=VERTEX_POINT('',#42883);
#12043=VERTEX_POINT('',#42885);
#12044=VERTEX_POINT('',#42887);
#12045=VERTEX_POINT('',#42889);
#12046=VERTEX_POINT('',#42891);
#12047=VERTEX_POINT('',#42895);
#12048=VERTEX_POINT('',#42897);
#12049=VERTEX_POINT('',#42899);
#12050=VERTEX_POINT('',#42901);
#12051=VERTEX_POINT('',#42905);
#12052=VERTEX_POINT('',#42909);
#12053=VERTEX_POINT('',#42911);
#12054=VERTEX_POINT('',#42913);
#12055=VERTEX_POINT('',#42917);
#12056=VERTEX_POINT('',#42919);
#12057=VERTEX_POINT('',#42923);
#12058=VERTEX_POINT('',#42925);
#12059=VERTEX_POINT('',#42929);
#12060=VERTEX_POINT('',#42933);
#12061=VERTEX_POINT('',#42935);
#12062=VERTEX_POINT('',#42939);
#12063=VERTEX_POINT('',#42941);
#12064=VERTEX_POINT('',#42945);
#12065=VERTEX_POINT('',#42947);
#12066=VERTEX_POINT('',#42951);
#12067=VERTEX_POINT('',#42955);
#12068=VERTEX_POINT('',#42959);
#12069=VERTEX_POINT('',#42960);
#12070=VERTEX_POINT('',#42962);
#12071=VERTEX_POINT('',#42964);
#12072=VERTEX_POINT('',#42971);
#12073=VERTEX_POINT('',#42975);
#12074=VERTEX_POINT('',#42979);
#12075=VERTEX_POINT('',#42980);
#12076=VERTEX_POINT('',#42982);
#12077=VERTEX_POINT('',#42987);
#12078=VERTEX_POINT('',#42991);
#12079=VERTEX_POINT('',#42997);
#12080=VERTEX_POINT('',#43001);
#12081=VERTEX_POINT('',#43008);
#12082=VERTEX_POINT('',#43013);
#12083=VERTEX_POINT('',#43015);
#12084=VERTEX_POINT('',#43017);
#12085=VERTEX_POINT('',#43019);
#12086=VERTEX_POINT('',#43021);
#12087=VERTEX_POINT('',#43023);
#12088=VERTEX_POINT('',#43025);
#12089=VERTEX_POINT('',#43027);
#12090=VERTEX_POINT('',#43029);
#12091=VERTEX_POINT('',#43031);
#12092=VERTEX_POINT('',#43033);
#12093=VERTEX_POINT('',#43037);
#12094=VERTEX_POINT('',#43039);
#12095=VERTEX_POINT('',#43041);
#12096=VERTEX_POINT('',#43045);
#12097=VERTEX_POINT('',#43050);
#12098=VERTEX_POINT('',#43054);
#12099=VERTEX_POINT('',#43058);
#12100=VERTEX_POINT('',#43062);
#12101=VERTEX_POINT('',#43063);
#12102=VERTEX_POINT('',#43065);
#12103=VERTEX_POINT('',#43070);
#12104=VERTEX_POINT('',#43074);
#12105=VERTEX_POINT('',#43076);
#12106=VERTEX_POINT('',#43080);
#12107=VERTEX_POINT('',#43081);
#12108=VERTEX_POINT('',#43084);
#12109=VERTEX_POINT('',#43090);
#12110=VERTEX_POINT('',#43091);
#12111=VERTEX_POINT('',#43099);
#12112=VERTEX_POINT('',#43104);
#12113=VERTEX_POINT('',#43106);
#12114=VERTEX_POINT('',#43110);
#12115=VERTEX_POINT('',#43112);
#12116=VERTEX_POINT('',#43114);
#12117=VERTEX_POINT('',#43119);
#12118=VERTEX_POINT('',#43120);
#12119=VERTEX_POINT('',#43122);
#12120=VERTEX_POINT('',#43124);
#12121=VERTEX_POINT('',#43128);
#12122=VERTEX_POINT('',#43130);
#12123=VERTEX_POINT('',#43134);
#12124=VERTEX_POINT('',#43136);
#12125=VERTEX_POINT('',#43138);
#12126=VERTEX_POINT('',#43142);
#12127=VERTEX_POINT('',#43143);
#12128=VERTEX_POINT('',#43145);
#12129=VERTEX_POINT('',#43148);
#12130=VERTEX_POINT('',#43152);
#12131=VERTEX_POINT('',#43154);
#12132=VERTEX_POINT('',#43160);
#12133=VERTEX_POINT('',#43161);
#12134=VERTEX_POINT('',#43163);
#12135=VERTEX_POINT('',#43165);
#12136=VERTEX_POINT('',#43173);
#12137=VERTEX_POINT('',#43179);
#12138=VERTEX_POINT('',#43181);
#12139=VERTEX_POINT('',#43183);
#12140=VERTEX_POINT('',#43185);
#12141=VERTEX_POINT('',#43187);
#12142=VERTEX_POINT('',#43189);
#12143=VERTEX_POINT('',#43197);
#12144=VERTEX_POINT('',#43198);
#12145=VERTEX_POINT('',#43203);
#12146=VERTEX_POINT('',#43207);
#12147=VERTEX_POINT('',#43208);
#12148=VERTEX_POINT('',#43214);
#12149=VERTEX_POINT('',#43220);
#12150=VERTEX_POINT('',#43222);
#12151=VERTEX_POINT('',#43229);
#12152=VERTEX_POINT('',#43231);
#12153=VERTEX_POINT('',#43233);
#12154=VERTEX_POINT('',#43241);
#12155=VERTEX_POINT('',#43245);
#12156=VERTEX_POINT('',#43248);
#12157=VERTEX_POINT('',#43249);
#12158=VERTEX_POINT('',#43251);
#12159=VERTEX_POINT('',#43253);
#12160=VERTEX_POINT('',#43257);
#12161=VERTEX_POINT('',#43259);
#12162=VERTEX_POINT('',#43265);
#12163=VERTEX_POINT('',#43272);
#12164=VERTEX_POINT('',#43273);
#12165=VERTEX_POINT('',#43275);
#12166=VERTEX_POINT('',#43277);
#12167=VERTEX_POINT('',#43281);
#12168=VERTEX_POINT('',#43283);
#12169=VERTEX_POINT('',#43287);
#12170=VERTEX_POINT('',#43291);
#12171=VERTEX_POINT('',#43297);
#12172=VERTEX_POINT('',#43299);
#12173=VERTEX_POINT('',#43303);
#12174=VERTEX_POINT('',#43310);
#12175=VERTEX_POINT('',#43320);
#12176=VERTEX_POINT('',#43322);
#12177=VERTEX_POINT('',#43326);
#12178=VERTEX_POINT('',#43330);
#12179=VERTEX_POINT('',#43336);
#12180=VERTEX_POINT('',#43338);
#12181=VERTEX_POINT('',#43342);
#12182=VERTEX_POINT('',#43349);
#15009=EDGE_CURVE('',#12011,#12012,#7065,.F.);
#15010=EDGE_CURVE('',#12012,#12013,#7066,.T.);
#15011=EDGE_CURVE('',#12013,#12014,#7067,.F.);
#15012=EDGE_CURVE('',#12014,#12011,#7068,.T.);
#15013=EDGE_CURVE('',#12015,#12012,#7069,.T.);
#15014=EDGE_CURVE('',#12016,#12015,#7070,.T.);
#15015=EDGE_CURVE('',#12013,#12016,#7071,.T.);
#15016=EDGE_CURVE('',#12017,#12018,#7072,.T.);
#15017=EDGE_CURVE('',#12018,#12019,#7073,.T.);
#15018=EDGE_CURVE('',#12019,#12020,#7074,.T.);
#15019=EDGE_CURVE('',#12020,#12021,#7075,.T.);
#15020=EDGE_CURVE('',#12021,#12022,#7076,.T.);
#15021=EDGE_CURVE('',#12022,#12017,#7077,.T.);
#15022=EDGE_CURVE('',#12023,#12021,#7078,.T.);
#15023=EDGE_CURVE('',#12024,#12023,#7079,.T.);
#15024=EDGE_CURVE('',#12022,#12024,#7080,.T.);
#15025=EDGE_CURVE('',#12025,#12020,#7081,.T.);
#15026=EDGE_CURVE('',#12025,#12026,#7082,.T.);
#15027=EDGE_CURVE('',#12027,#12026,#7083,.T.);
#15028=EDGE_CURVE('',#12023,#12027,#7084,.T.);
#15029=EDGE_CURVE('',#12019,#12028,#7085,.T.);
#15030=EDGE_CURVE('',#12029,#12028,#7086,.T.);
#15031=EDGE_CURVE('',#12030,#12029,#7087,.T.);
#15032=EDGE_CURVE('',#12030,#12025,#7088,.T.);
#15033=EDGE_CURVE('',#12031,#12032,#7089,.F.);
#15034=EDGE_CURVE('',#12032,#12033,#7090,.T.);
#15035=EDGE_CURVE('',#12033,#12034,#7091,.F.);
#15036=EDGE_CURVE('',#12034,#12031,#7092,.T.);
#15037=EDGE_CURVE('',#12033,#12014,#7093,.T.);
#15038=EDGE_CURVE('',#12011,#12032,#7094,.T.);
#15039=EDGE_CURVE('',#12035,#12036,#7095,.F.);
#15040=EDGE_CURVE('',#12036,#12037,#7096,.T.);
#15041=EDGE_CURVE('',#12037,#12038,#7097,.F.);
#15042=EDGE_CURVE('',#12038,#12035,#7098,.T.);
#15043=EDGE_CURVE('',#12039,#12036,#7099,.T.);
#15044=EDGE_CURVE('',#12040,#12039,#7100,.T.);
#15045=EDGE_CURVE('',#12037,#12040,#7101,.T.);
#15046=EDGE_CURVE('',#12041,#12042,#7102,.T.);
#15047=EDGE_CURVE('',#12042,#12043,#7103,.T.);
#15048=EDGE_CURVE('',#12043,#12044,#7104,.T.);
#15049=EDGE_CURVE('',#12044,#12045,#7105,.T.);
#15050=EDGE_CURVE('',#12045,#12046,#7106,.T.);
#15051=EDGE_CURVE('',#12046,#12041,#7107,.T.);
#15052=EDGE_CURVE('',#12046,#12047,#7108,.T.);
#15053=EDGE_CURVE('',#12048,#12047,#7109,.T.);
#15054=EDGE_CURVE('',#12049,#12048,#7110,.T.);
#15055=EDGE_CURVE('',#12049,#12050,#7111,.T.);
#15056=EDGE_CURVE('',#12041,#12050,#7112,.T.);
#15057=EDGE_CURVE('',#12051,#12045,#7113,.T.);
#15058=EDGE_CURVE('',#12047,#12051,#7114,.T.);
#15059=EDGE_CURVE('',#12052,#12044,#7115,.T.);
#15060=EDGE_CURVE('',#12052,#12053,#7116,.T.);
#15061=EDGE_CURVE('',#12054,#12053,#7117,.T.);
#15062=EDGE_CURVE('',#12051,#12054,#7118,.T.);
#15063=EDGE_CURVE('',#12054,#12055,#7119,.T.);
#15064=EDGE_CURVE('',#12055,#12056,#7120,.T.);
#15065=EDGE_CURVE('',#12056,#12048,#7121,.T.);
#15066=EDGE_CURVE('',#12056,#12057,#7122,.T.);
#15067=EDGE_CURVE('',#12057,#12058,#7123,.T.);
#15068=EDGE_CURVE('',#12058,#12049,#7124,.T.);
#15069=EDGE_CURVE('',#12059,#12055,#7125,.T.);
#15070=EDGE_CURVE('',#12057,#12059,#7126,.T.);
#15071=EDGE_CURVE('',#12053,#12060,#7127,.T.);
#15072=EDGE_CURVE('',#12060,#12061,#7128,.T.);
#15073=EDGE_CURVE('',#12059,#12061,#7129,.T.);
#15074=EDGE_CURVE('',#12050,#12062,#7130,.T.);
#15075=EDGE_CURVE('',#12062,#12063,#7131,.T.);
#15076=EDGE_CURVE('',#12063,#12042,#7132,.T.);
#15077=EDGE_CURVE('',#12062,#12064,#7133,.T.);
#15078=EDGE_CURVE('',#12064,#12065,#7134,.F.);
#15079=EDGE_CURVE('',#12065,#12063,#7135,.T.);
#15080=EDGE_CURVE('',#12066,#12063,#7136,.T.);
#15081=EDGE_CURVE('',#12043,#12066,#7137,.T.);
#15082=EDGE_CURVE('',#12067,#12065,#7138,.T.);
#15083=EDGE_CURVE('',#12066,#12067,#7139,.T.);
#15084=EDGE_CURVE('',#12068,#12069,#7140,.F.);
#15085=EDGE_CURVE('',#12069,#12070,#7141,.T.);
#15086=EDGE_CURVE('',#12070,#12071,#7142,.F.);
#15087=EDGE_CURVE('',#12071,#12068,#7143,.T.);
#15088=EDGE_CURVE('',#12070,#12038,#7144,.T.);
#15089=EDGE_CURVE('',#12035,#12069,#7145,.T.);
#15090=EDGE_CURVE('',#12072,#12057,#7146,.T.);
#15091=EDGE_CURVE('',#12058,#12072,#7147,.T.);
#15092=EDGE_CURVE('',#12061,#12073,#7148,.T.);
#15093=EDGE_CURVE('',#12073,#12072,#7149,.T.);
#15094=EDGE_CURVE('',#12074,#12075,#7150,.T.);
#15095=EDGE_CURVE('',#12076,#12074,#7151,.T.);
#15096=EDGE_CURVE('',#12075,#12076,#7152,.T.);
#15097=EDGE_CURVE('',#12028,#12076,#7153,.T.);
#15098=EDGE_CURVE('',#12074,#12077,#7154,.T.);
#15099=EDGE_CURVE('',#12077,#12029,#7155,.T.);
#15100=EDGE_CURVE('',#12017,#12078,#7156,.T.);
#15101=EDGE_CURVE('',#12078,#12075,#7157,.T.);
#15102=EDGE_CURVE('',#12076,#12018,#7158,.T.);
#15103=EDGE_CURVE('',#12015,#12074,#7159,.T.);
#15104=EDGE_CURVE('',#12075,#12079,#7160,.T.);
#15105=EDGE_CURVE('',#12079,#12015,#7161,.T.);
#15106=EDGE_CURVE('',#12079,#12080,#7162,.T.);
#15107=EDGE_CURVE('',#12080,#12016,#7163,.T.);
#15108=EDGE_CURVE('',#12080,#12058,#7164,.T.);
#15109=EDGE_CURVE('',#12072,#12016,#7165,.T.);
#15110=EDGE_CURVE('',#12060,#12081,#7166,.T.);
#15111=EDGE_CURVE('',#12081,#12039,#7167,.T.);
#15112=EDGE_CURVE('',#12039,#12073,#7168,.T.);
#15113=EDGE_CURVE('',#12082,#12078,#7169,.T.);
#15114=EDGE_CURVE('',#12083,#12082,#7170,.T.);
#15115=EDGE_CURVE('',#12084,#12083,#7171,.T.);
#15116=EDGE_CURVE('',#12085,#12084,#7172,.T.);
#15117=EDGE_CURVE('',#12086,#12085,#7173,.T.);
#15118=EDGE_CURVE('',#12087,#12086,#7174,.T.);
#15119=EDGE_CURVE('',#12088,#12087,#7175,.T.);
#15120=EDGE_CURVE('',#12089,#12088,#7176,.T.);
#15121=EDGE_CURVE('',#12090,#12089,#7177,.T.);
#15122=EDGE_CURVE('',#12091,#12090,#7178,.T.);
#15123=EDGE_CURVE('',#12092,#12091,#7179,.T.);
#15124=EDGE_CURVE('',#12064,#12092,#7180,.T.);
#15125=EDGE_CURVE('',#12093,#12024,#7181,.T.);
#15126=EDGE_CURVE('',#12027,#12094,#7182,.T.);
#15127=EDGE_CURVE('',#12094,#12095,#7183,.T.);
#15128=EDGE_CURVE('',#12095,#12093,#7184,.T.);
#15129=EDGE_CURVE('',#12095,#12096,#7185,.T.);
#15130=EDGE_CURVE('',#12083,#12096,#7186,.T.);
#15131=EDGE_CURVE('',#12082,#12093,#7187,.T.);
#15132=EDGE_CURVE('',#12097,#12094,#7188,.T.);
#15133=EDGE_CURVE('',#12097,#12096,#7189,.T.);
#15134=EDGE_CURVE('',#12026,#12098,#7190,.T.);
#15135=EDGE_CURVE('',#12098,#12097,#7191,.T.);
#15136=EDGE_CURVE('',#12096,#12099,#7192,.T.);
#15137=EDGE_CURVE('',#12099,#12084,#7193,.F.);
#15138=EDGE_CURVE('',#12100,#12101,#7194,.T.);
#15139=EDGE_CURVE('',#12101,#12102,#7195,.T.);
#15140=EDGE_CURVE('',#12102,#12090,#7196,.T.);
#15141=EDGE_CURVE('',#12089,#12100,#7197,.T.);
#15142=EDGE_CURVE('',#12088,#12103,#7198,.T.);
#15143=EDGE_CURVE('',#12103,#12100,#7199,.T.);
#15144=EDGE_CURVE('',#12104,#12087,#7200,.T.);
#15145=EDGE_CURVE('',#12105,#12104,#7201,.T.);
#15146=EDGE_CURVE('',#12087,#12105,#7202,.T.);
#15147=EDGE_CURVE('',#12106,#12107,#7203,.T.);
#15148=EDGE_CURVE('',#12107,#12105,#7204,.T.);
#15149=EDGE_CURVE('',#12104,#12108,#7205,.T.);
#15150=EDGE_CURVE('',#12108,#12106,#7206,.T.);
#15151=EDGE_CURVE('',#12105,#12103,#7207,.T.);
#15152=EDGE_CURVE('',#12109,#12110,#7208,.T.);
#15153=EDGE_CURVE('',#12110,#12104,#7209,.T.);
#15154=EDGE_CURVE('',#12086,#12109,#7210,.T.);
#15155=EDGE_CURVE('',#12100,#12034,#7211,.T.);
#15156=EDGE_CURVE('',#12031,#12103,#7212,.T.);
#15157=EDGE_CURVE('',#12111,#12107,#7213,.T.);
#15158=EDGE_CURVE('',#12111,#12071,#7214,.T.);
#15159=EDGE_CURVE('',#12077,#12040,#7215,.T.);
#15160=EDGE_CURVE('',#12112,#12106,#7216,.T.);
#15161=EDGE_CURVE('',#12112,#12113,#7217,.T.);
#15162=EDGE_CURVE('',#12113,#12111,#7218,.T.);
#15163=EDGE_CURVE('',#12108,#12114,#7219,.T.);
#15164=EDGE_CURVE('',#12115,#12114,#7220,.T.);
#15165=EDGE_CURVE('',#12115,#12116,#7221,.T.);
#15166=EDGE_CURVE('',#12116,#12112,#7222,.T.);
#15167=EDGE_CURVE('',#12114,#12110,#7223,.T.);
#15168=EDGE_CURVE('',#12117,#12118,#7224,.T.);
#15169=EDGE_CURVE('',#12119,#12117,#2214,.T.);
#15170=EDGE_CURVE('',#12120,#12119,#7225,.T.);
#15171=EDGE_CURVE('',#12118,#12120,#2215,.T.);
#15172=EDGE_CURVE('',#12109,#12121,#7226,.T.);
#15173=EDGE_CURVE('',#12121,#12122,#7227,.T.);
#15174=EDGE_CURVE('',#12122,#12115,#7228,.T.);
#15175=EDGE_CURVE('',#12122,#12123,#7229,.T.);
#15176=EDGE_CURVE('',#12124,#12123,#7230,.T.);
#15177=EDGE_CURVE('',#12125,#12124,#7231,.T.);
#15178=EDGE_CURVE('',#12125,#12116,#7232,.T.);
#15179=EDGE_CURVE('',#12126,#12127,#7233,.T.);
#15180=EDGE_CURVE('',#12127,#12128,#7234,.T.);
#15181=EDGE_CURVE('',#12128,#12124,#7235,.T.);
#15182=EDGE_CURVE('',#12123,#12129,#7236,.T.);
#15183=EDGE_CURVE('',#12129,#12126,#7237,.T.);
#15184=EDGE_CURVE('',#12128,#12130,#7238,.T.);
#15185=EDGE_CURVE('',#12131,#12130,#7239,.T.);
#15186=EDGE_CURVE('',#12131,#12125,#7240,.T.);
#15187=EDGE_CURVE('',#12099,#12127,#7241,.T.);
#15188=EDGE_CURVE('',#12130,#12099,#7242,.T.);
#15189=EDGE_CURVE('',#12132,#12133,#7243,.T.);
#15190=EDGE_CURVE('',#12134,#12132,#2216,.T.);
#15191=EDGE_CURVE('',#12135,#12134,#7244,.T.);
#15192=EDGE_CURVE('',#12133,#12135,#2217,.T.);
#15193=EDGE_CURVE('',#12126,#12085,#7245,.T.);
#15194=EDGE_CURVE('',#12129,#12121,#7246,.T.);
#15195=EDGE_CURVE('',#12081,#12136,#7247,.T.);
#15196=EDGE_CURVE('',#12136,#12040,#7248,.T.);
#15197=EDGE_CURVE('',#12136,#12030,#7249,.T.);
#15198=EDGE_CURVE('',#12137,#12052,#7250,.T.);
#15199=EDGE_CURVE('',#12138,#12137,#7251,.T.);
#15200=EDGE_CURVE('',#12139,#12138,#7252,.T.);
#15201=EDGE_CURVE('',#12140,#12139,#7253,.T.);
#15202=EDGE_CURVE('',#12141,#12140,#7254,.T.);
#15203=EDGE_CURVE('',#12142,#12141,#7255,.T.);
#15204=EDGE_CURVE('',#12113,#12142,#7256,.T.);
#15205=EDGE_CURVE('',#12098,#12131,#7257,.T.);
#15206=EDGE_CURVE('',#12130,#12097,#7258,.T.);
#15207=EDGE_CURVE('',#12143,#12144,#7259,.T.);
#15208=EDGE_CURVE('',#12141,#12143,#7260,.T.);
#15209=EDGE_CURVE('',#12144,#12141,#7261,.T.);
#15210=EDGE_CURVE('',#12143,#12145,#7262,.T.);
#15211=EDGE_CURVE('',#12145,#12142,#7263,.T.);
#15212=EDGE_CURVE('',#12146,#12147,#7264,.T.);
#15213=EDGE_CURVE('',#12147,#12144,#7265,.T.);
#15214=EDGE_CURVE('',#12140,#12146,#7266,.T.);
#15215=EDGE_CURVE('',#12101,#12143,#7267,.T.);
#15216=EDGE_CURVE('',#12144,#12148,#7268,.T.);
#15217=EDGE_CURVE('',#12148,#12102,#7269,.T.);
#15218=EDGE_CURVE('',#12145,#12111,#7270,.T.);
#15219=EDGE_CURVE('',#12148,#12149,#7271,.T.);
#15220=EDGE_CURVE('',#12149,#12150,#7272,.T.);
#15221=EDGE_CURVE('',#12150,#12091,#7273,.T.);
#15222=EDGE_CURVE('',#12068,#12145,#7274,.T.);
#15223=EDGE_CURVE('',#12151,#12150,#7275,.T.);
#15224=EDGE_CURVE('',#12151,#12152,#7276,.T.);
#15225=EDGE_CURVE('',#12153,#12152,#7277,.T.);
#15226=EDGE_CURVE('',#12092,#12153,#7278,.T.);
#15227=EDGE_CURVE('',#12067,#12138,#7279,.F.);
#15228=EDGE_CURVE('',#12137,#12066,#7280,.T.);
#15229=EDGE_CURVE('',#12153,#12154,#7281,.T.);
#15230=EDGE_CURVE('',#12154,#12065,#7282,.T.);
#15231=EDGE_CURVE('',#12155,#12154,#7283,.T.);
#15232=EDGE_CURVE('',#12067,#12155,#7284,.T.);
#15233=EDGE_CURVE('',#12156,#12157,#7285,.T.);
#15234=EDGE_CURVE('',#12158,#12156,#2218,.T.);
#15235=EDGE_CURVE('',#12159,#12158,#7286,.T.);
#15236=EDGE_CURVE('',#12157,#12159,#2219,.T.);
#15237=EDGE_CURVE('',#12152,#12160,#7287,.T.);
#15238=EDGE_CURVE('',#12160,#12161,#7288,.T.);
#15239=EDGE_CURVE('',#12155,#12161,#7289,.T.);
#15240=EDGE_CURVE('',#12161,#12139,#7290,.T.);
#15241=EDGE_CURVE('',#12160,#12162,#7291,.T.);
#15242=EDGE_CURVE('',#12146,#12162,#7292,.T.);
#15243=EDGE_CURVE('',#12162,#12151,#7293,.T.);
#15244=EDGE_CURVE('',#12149,#12147,#7294,.T.);
#15245=EDGE_CURVE('',#12163,#12164,#7295,.T.);
#15246=EDGE_CURVE('',#12165,#12163,#2220,.T.);
#15247=EDGE_CURVE('',#12166,#12165,#7296,.T.);
#15248=EDGE_CURVE('',#12164,#12166,#2221,.T.);
#15249=EDGE_CURVE('',#12167,#12132,#7297,.T.);
#15250=EDGE_CURVE('',#12133,#12168,#7298,.T.);
#15251=EDGE_CURVE('',#12168,#12167,#7299,.T.);
#15252=EDGE_CURVE('',#12169,#12134,#7300,.T.);
#15253=EDGE_CURVE('',#12167,#12169,#2222,.T.);
#15254=EDGE_CURVE('',#12170,#12135,#7301,.T.);
#15255=EDGE_CURVE('',#12169,#12170,#7302,.T.);
#15256=EDGE_CURVE('',#12170,#12168,#2223,.T.);
#15257=EDGE_CURVE('',#12171,#12167,#7303,.T.);
#15258=EDGE_CURVE('',#12172,#12171,#2224,.T.);
#15259=EDGE_CURVE('',#12172,#12169,#7304,.T.);
#15260=EDGE_CURVE('',#12173,#12168,#7305,.T.);
#15261=EDGE_CURVE('',#12171,#12173,#7306,.T.);
#15262=EDGE_CURVE('',#12173,#12117,#7307,.T.);
#15263=EDGE_CURVE('',#12118,#12171,#7308,.T.);
#15264=EDGE_CURVE('',#12174,#12119,#7309,.T.);
#15265=EDGE_CURVE('',#12173,#12174,#2225,.T.);
#15266=EDGE_CURVE('',#12172,#12120,#7310,.T.);
#15267=EDGE_CURVE('',#12174,#12172,#7311,.T.);
#15268=EDGE_CURVE('',#12174,#12170,#7312,.T.);
#15269=EDGE_CURVE('',#12175,#12156,#7313,.T.);
#15270=EDGE_CURVE('',#12157,#12176,#7314,.T.);
#15271=EDGE_CURVE('',#12176,#12175,#7315,.T.);
#15272=EDGE_CURVE('',#12177,#12158,#7316,.T.);
#15273=EDGE_CURVE('',#12175,#12177,#2226,.T.);
#15274=EDGE_CURVE('',#12178,#12159,#7317,.T.);
#15275=EDGE_CURVE('',#12177,#12178,#7318,.T.);
#15276=EDGE_CURVE('',#12178,#12176,#2227,.T.);
#15277=EDGE_CURVE('',#12179,#12175,#7319,.T.);
#15278=EDGE_CURVE('',#12180,#12179,#2228,.T.);
#15279=EDGE_CURVE('',#12180,#12177,#7320,.T.);
#15280=EDGE_CURVE('',#12181,#12176,#7321,.T.);
#15281=EDGE_CURVE('',#12179,#12181,#7322,.T.);
#15282=EDGE_CURVE('',#12181,#12163,#7323,.T.);
#15283=EDGE_CURVE('',#12164,#12179,#7324,.T.);
#15284=EDGE_CURVE('',#12182,#12165,#7325,.T.);
#15285=EDGE_CURVE('',#12181,#12182,#2229,.T.);
#15286=EDGE_CURVE('',#12180,#12166,#7326,.T.);
#15287=EDGE_CURVE('',#12182,#12180,#7327,.T.);
#15288=EDGE_CURVE('',#12182,#12178,#7328,.T.);
#20251=ORIENTED_EDGE('',*,*,#15009,.T.);
#20252=ORIENTED_EDGE('',*,*,#15010,.T.);
#20253=ORIENTED_EDGE('',*,*,#15011,.T.);
#20254=ORIENTED_EDGE('',*,*,#15012,.T.);
#20255=ORIENTED_EDGE('',*,*,#15010,.F.);
#20256=ORIENTED_EDGE('',*,*,#15013,.F.);
#20257=ORIENTED_EDGE('',*,*,#15014,.F.);
#20258=ORIENTED_EDGE('',*,*,#15015,.F.);
#20259=ORIENTED_EDGE('',*,*,#15016,.T.);
#20260=ORIENTED_EDGE('',*,*,#15017,.T.);
#20261=ORIENTED_EDGE('',*,*,#15018,.T.);
#20262=ORIENTED_EDGE('',*,*,#15019,.T.);
#20263=ORIENTED_EDGE('',*,*,#15020,.T.);
#20264=ORIENTED_EDGE('',*,*,#15021,.T.);
#20265=ORIENTED_EDGE('',*,*,#15020,.F.);
#20266=ORIENTED_EDGE('',*,*,#15022,.F.);
#20267=ORIENTED_EDGE('',*,*,#15023,.F.);
#20268=ORIENTED_EDGE('',*,*,#15024,.F.);
#20269=ORIENTED_EDGE('',*,*,#15019,.F.);
#20270=ORIENTED_EDGE('',*,*,#15025,.F.);
#20271=ORIENTED_EDGE('',*,*,#15026,.T.);
#20272=ORIENTED_EDGE('',*,*,#15027,.F.);
#20273=ORIENTED_EDGE('',*,*,#15028,.F.);
#20274=ORIENTED_EDGE('',*,*,#15022,.T.);
#20275=ORIENTED_EDGE('',*,*,#15018,.F.);
#20276=ORIENTED_EDGE('',*,*,#15029,.T.);
#20277=ORIENTED_EDGE('',*,*,#15030,.F.);
#20278=ORIENTED_EDGE('',*,*,#15031,.F.);
#20279=ORIENTED_EDGE('',*,*,#15032,.T.);
#20280=ORIENTED_EDGE('',*,*,#15025,.T.);
#20281=ORIENTED_EDGE('',*,*,#15033,.T.);
#20282=ORIENTED_EDGE('',*,*,#15034,.T.);
#20283=ORIENTED_EDGE('',*,*,#15035,.T.);
#20284=ORIENTED_EDGE('',*,*,#15036,.T.);
#20285=ORIENTED_EDGE('',*,*,#15012,.F.);
#20286=ORIENTED_EDGE('',*,*,#15037,.F.);
#20287=ORIENTED_EDGE('',*,*,#15034,.F.);
#20288=ORIENTED_EDGE('',*,*,#15038,.F.);
#20289=ORIENTED_EDGE('',*,*,#15039,.T.);
#20290=ORIENTED_EDGE('',*,*,#15040,.T.);
#20291=ORIENTED_EDGE('',*,*,#15041,.T.);
#20292=ORIENTED_EDGE('',*,*,#15042,.T.);
#20293=ORIENTED_EDGE('',*,*,#15040,.F.);
#20294=ORIENTED_EDGE('',*,*,#15043,.F.);
#20295=ORIENTED_EDGE('',*,*,#15044,.F.);
#20296=ORIENTED_EDGE('',*,*,#15045,.F.);
#20297=ORIENTED_EDGE('',*,*,#15046,.T.);
#20298=ORIENTED_EDGE('',*,*,#15047,.T.);
#20299=ORIENTED_EDGE('',*,*,#15048,.T.);
#20300=ORIENTED_EDGE('',*,*,#15049,.T.);
#20301=ORIENTED_EDGE('',*,*,#15050,.T.);
#20302=ORIENTED_EDGE('',*,*,#15051,.T.);
#20303=ORIENTED_EDGE('',*,*,#15051,.F.);
#20304=ORIENTED_EDGE('',*,*,#15052,.T.);
#20305=ORIENTED_EDGE('',*,*,#15053,.F.);
#20306=ORIENTED_EDGE('',*,*,#15054,.F.);
#20307=ORIENTED_EDGE('',*,*,#15055,.T.);
#20308=ORIENTED_EDGE('',*,*,#15056,.F.);
#20309=ORIENTED_EDGE('',*,*,#15050,.F.);
#20310=ORIENTED_EDGE('',*,*,#15057,.F.);
#20311=ORIENTED_EDGE('',*,*,#15058,.F.);
#20312=ORIENTED_EDGE('',*,*,#15052,.F.);
#20313=ORIENTED_EDGE('',*,*,#15049,.F.);
#20314=ORIENTED_EDGE('',*,*,#15059,.F.);
#20315=ORIENTED_EDGE('',*,*,#15060,.T.);
#20316=ORIENTED_EDGE('',*,*,#15061,.F.);
#20317=ORIENTED_EDGE('',*,*,#15062,.F.);
#20318=ORIENTED_EDGE('',*,*,#15057,.T.);
#20319=ORIENTED_EDGE('',*,*,#15053,.T.);
#20320=ORIENTED_EDGE('',*,*,#15058,.T.);
#20321=ORIENTED_EDGE('',*,*,#15062,.T.);
#20322=ORIENTED_EDGE('',*,*,#15063,.T.);
#20323=ORIENTED_EDGE('',*,*,#15064,.T.);
#20324=ORIENTED_EDGE('',*,*,#15065,.T.);
#20325=ORIENTED_EDGE('',*,*,#15065,.F.);
#20326=ORIENTED_EDGE('',*,*,#15066,.T.);
#20327=ORIENTED_EDGE('',*,*,#15067,.T.);
#20328=ORIENTED_EDGE('',*,*,#15068,.T.);
#20329=ORIENTED_EDGE('',*,*,#15054,.T.);
#20330=ORIENTED_EDGE('',*,*,#15064,.F.);
#20331=ORIENTED_EDGE('',*,*,#15069,.F.);
#20332=ORIENTED_EDGE('',*,*,#15070,.F.);
#20333=ORIENTED_EDGE('',*,*,#15066,.F.);
#20334=ORIENTED_EDGE('',*,*,#15063,.F.);
#20335=ORIENTED_EDGE('',*,*,#15061,.T.);
#20336=ORIENTED_EDGE('',*,*,#15071,.T.);
#20337=ORIENTED_EDGE('',*,*,#15072,.T.);
#20338=ORIENTED_EDGE('',*,*,#15073,.F.);
#20339=ORIENTED_EDGE('',*,*,#15069,.T.);
#20340=ORIENTED_EDGE('',*,*,#15046,.F.);
#20341=ORIENTED_EDGE('',*,*,#15056,.T.);
#20342=ORIENTED_EDGE('',*,*,#15074,.T.);
#20343=ORIENTED_EDGE('',*,*,#15075,.T.);
#20344=ORIENTED_EDGE('',*,*,#15076,.T.);
#20345=ORIENTED_EDGE('',*,*,#15077,.T.);
#20346=ORIENTED_EDGE('',*,*,#15078,.T.);
#20347=ORIENTED_EDGE('',*,*,#15079,.T.);
#20348=ORIENTED_EDGE('',*,*,#15075,.F.);
#20349=ORIENTED_EDGE('',*,*,#15047,.F.);
#20350=ORIENTED_EDGE('',*,*,#15076,.F.);
#20351=ORIENTED_EDGE('',*,*,#15080,.F.);
#20352=ORIENTED_EDGE('',*,*,#15081,.F.);
#20353=ORIENTED_EDGE('',*,*,#15079,.F.);
#20354=ORIENTED_EDGE('',*,*,#15082,.F.);
#20355=ORIENTED_EDGE('',*,*,#15083,.F.);
#20356=ORIENTED_EDGE('',*,*,#15080,.T.);
#20357=ORIENTED_EDGE('',*,*,#15084,.T.);
#20358=ORIENTED_EDGE('',*,*,#15085,.T.);
#20359=ORIENTED_EDGE('',*,*,#15086,.T.);
#20360=ORIENTED_EDGE('',*,*,#15087,.T.);
#20361=ORIENTED_EDGE('',*,*,#15042,.F.);
#20362=ORIENTED_EDGE('',*,*,#15088,.F.);
#20363=ORIENTED_EDGE('',*,*,#15085,.F.);
#20364=ORIENTED_EDGE('',*,*,#15089,.F.);
#20365=ORIENTED_EDGE('',*,*,#15067,.F.);
#20366=ORIENTED_EDGE('',*,*,#15090,.F.);
#20367=ORIENTED_EDGE('',*,*,#15091,.F.);
#20368=ORIENTED_EDGE('',*,*,#15092,.T.);
#20369=ORIENTED_EDGE('',*,*,#15093,.T.);
#20370=ORIENTED_EDGE('',*,*,#15090,.T.);
#20371=ORIENTED_EDGE('',*,*,#15070,.T.);
#20372=ORIENTED_EDGE('',*,*,#15073,.T.);
#20373=ORIENTED_EDGE('',*,*,#15094,.F.);
#20374=ORIENTED_EDGE('',*,*,#15095,.F.);
#20375=ORIENTED_EDGE('',*,*,#15096,.F.);
#20376=ORIENTED_EDGE('',*,*,#15030,.T.);
#20377=ORIENTED_EDGE('',*,*,#15097,.T.);
#20378=ORIENTED_EDGE('',*,*,#15095,.T.);
#20379=ORIENTED_EDGE('',*,*,#15098,.T.);
#20380=ORIENTED_EDGE('',*,*,#15099,.T.);
#20381=ORIENTED_EDGE('',*,*,#15016,.F.);
#20382=ORIENTED_EDGE('',*,*,#15100,.T.);
#20383=ORIENTED_EDGE('',*,*,#15101,.T.);
#20384=ORIENTED_EDGE('',*,*,#15096,.T.);
#20385=ORIENTED_EDGE('',*,*,#15102,.T.);
#20386=ORIENTED_EDGE('',*,*,#15103,.T.);
#20387=ORIENTED_EDGE('',*,*,#15094,.T.);
#20388=ORIENTED_EDGE('',*,*,#15104,.T.);
#20389=ORIENTED_EDGE('',*,*,#15105,.T.);
#20390=ORIENTED_EDGE('',*,*,#15014,.T.);
#20391=ORIENTED_EDGE('',*,*,#15105,.F.);
#20392=ORIENTED_EDGE('',*,*,#15106,.T.);
#20393=ORIENTED_EDGE('',*,*,#15107,.T.);
#20394=ORIENTED_EDGE('',*,*,#15108,.T.);
#20395=ORIENTED_EDGE('',*,*,#15091,.T.);
#20396=ORIENTED_EDGE('',*,*,#15109,.T.);
#20397=ORIENTED_EDGE('',*,*,#15107,.F.);
#20398=ORIENTED_EDGE('',*,*,#15092,.F.);
#20399=ORIENTED_EDGE('',*,*,#15072,.F.);
#20400=ORIENTED_EDGE('',*,*,#15110,.T.);
#20401=ORIENTED_EDGE('',*,*,#15111,.T.);
#20402=ORIENTED_EDGE('',*,*,#15112,.T.);
#20403=ORIENTED_EDGE('',*,*,#15074,.F.);
#20404=ORIENTED_EDGE('',*,*,#15055,.F.);
#20405=ORIENTED_EDGE('',*,*,#15068,.F.);
#20406=ORIENTED_EDGE('',*,*,#15108,.F.);
#20407=ORIENTED_EDGE('',*,*,#15106,.F.);
#20408=ORIENTED_EDGE('',*,*,#15104,.F.);
#20409=ORIENTED_EDGE('',*,*,#15101,.F.);
#20410=ORIENTED_EDGE('',*,*,#15113,.F.);
#20411=ORIENTED_EDGE('',*,*,#15114,.F.);
#20412=ORIENTED_EDGE('',*,*,#15115,.F.);
#20413=ORIENTED_EDGE('',*,*,#15116,.F.);
#20414=ORIENTED_EDGE('',*,*,#15117,.F.);
#20415=ORIENTED_EDGE('',*,*,#15118,.F.);
#20416=ORIENTED_EDGE('',*,*,#15119,.F.);
#20417=ORIENTED_EDGE('',*,*,#15120,.F.);
#20418=ORIENTED_EDGE('',*,*,#15121,.F.);
#20419=ORIENTED_EDGE('',*,*,#15122,.F.);
#20420=ORIENTED_EDGE('',*,*,#15123,.F.);
#20421=ORIENTED_EDGE('',*,*,#15124,.F.);
#20422=ORIENTED_EDGE('',*,*,#15077,.F.);
#20423=ORIENTED_EDGE('',*,*,#15125,.T.);
#20424=ORIENTED_EDGE('',*,*,#15023,.T.);
#20425=ORIENTED_EDGE('',*,*,#15028,.T.);
#20426=ORIENTED_EDGE('',*,*,#15126,.T.);
#20427=ORIENTED_EDGE('',*,*,#15127,.T.);
#20428=ORIENTED_EDGE('',*,*,#15128,.T.);
#20429=ORIENTED_EDGE('',*,*,#15128,.F.);
#20430=ORIENTED_EDGE('',*,*,#15129,.T.);
#20431=ORIENTED_EDGE('',*,*,#15130,.F.);
#20432=ORIENTED_EDGE('',*,*,#15114,.T.);
#20433=ORIENTED_EDGE('',*,*,#15131,.T.);
#20434=ORIENTED_EDGE('',*,*,#15127,.F.);
#20435=ORIENTED_EDGE('',*,*,#15132,.F.);
#20436=ORIENTED_EDGE('',*,*,#15133,.T.);
#20437=ORIENTED_EDGE('',*,*,#15129,.F.);
#20438=ORIENTED_EDGE('',*,*,#15126,.F.);
#20439=ORIENTED_EDGE('',*,*,#15027,.T.);
#20440=ORIENTED_EDGE('',*,*,#15134,.T.);
#20441=ORIENTED_EDGE('',*,*,#15135,.T.);
#20442=ORIENTED_EDGE('',*,*,#15132,.T.);
#20443=ORIENTED_EDGE('',*,*,#15136,.T.);
#20444=ORIENTED_EDGE('',*,*,#15137,.T.);
#20445=ORIENTED_EDGE('',*,*,#15115,.T.);
#20446=ORIENTED_EDGE('',*,*,#15130,.T.);
#20447=ORIENTED_EDGE('',*,*,#15138,.T.);
#20448=ORIENTED_EDGE('',*,*,#15139,.T.);
#20449=ORIENTED_EDGE('',*,*,#15140,.T.);
#20450=ORIENTED_EDGE('',*,*,#15121,.T.);
#20451=ORIENTED_EDGE('',*,*,#15141,.T.);
#20452=ORIENTED_EDGE('',*,*,#15120,.T.);
#20453=ORIENTED_EDGE('',*,*,#15142,.T.);
#20454=ORIENTED_EDGE('',*,*,#15143,.T.);
#20455=ORIENTED_EDGE('',*,*,#15141,.F.);
#20456=ORIENTED_EDGE('',*,*,#15144,.F.);
#20457=ORIENTED_EDGE('',*,*,#15145,.F.);
#20458=ORIENTED_EDGE('',*,*,#15146,.F.);
#20459=ORIENTED_EDGE('',*,*,#15147,.T.);
#20460=ORIENTED_EDGE('',*,*,#15148,.T.);
#20461=ORIENTED_EDGE('',*,*,#15145,.T.);
#20462=ORIENTED_EDGE('',*,*,#15149,.T.);
#20463=ORIENTED_EDGE('',*,*,#15150,.T.);
#20464=ORIENTED_EDGE('',*,*,#15119,.T.);
#20465=ORIENTED_EDGE('',*,*,#15146,.T.);
#20466=ORIENTED_EDGE('',*,*,#15151,.T.);
#20467=ORIENTED_EDGE('',*,*,#15142,.F.);
#20468=ORIENTED_EDGE('',*,*,#15152,.T.);
#20469=ORIENTED_EDGE('',*,*,#15153,.T.);
#20470=ORIENTED_EDGE('',*,*,#15144,.T.);
#20471=ORIENTED_EDGE('',*,*,#15118,.T.);
#20472=ORIENTED_EDGE('',*,*,#15154,.T.);
#20473=ORIENTED_EDGE('',*,*,#15036,.F.);
#20474=ORIENTED_EDGE('',*,*,#15155,.F.);
#20475=ORIENTED_EDGE('',*,*,#15143,.F.);
#20476=ORIENTED_EDGE('',*,*,#15156,.F.);
#20477=ORIENTED_EDGE('',*,*,#15103,.F.);
#20478=ORIENTED_EDGE('',*,*,#15013,.T.);
#20479=ORIENTED_EDGE('',*,*,#15009,.F.);
#20480=ORIENTED_EDGE('',*,*,#15038,.T.);
#20481=ORIENTED_EDGE('',*,*,#15033,.F.);
#20482=ORIENTED_EDGE('',*,*,#15156,.T.);
#20483=ORIENTED_EDGE('',*,*,#15151,.F.);
#20484=ORIENTED_EDGE('',*,*,#15148,.F.);
#20485=ORIENTED_EDGE('',*,*,#15157,.F.);
#20486=ORIENTED_EDGE('',*,*,#15158,.T.);
#20487=ORIENTED_EDGE('',*,*,#15086,.F.);
#20488=ORIENTED_EDGE('',*,*,#15088,.T.);
#20489=ORIENTED_EDGE('',*,*,#15041,.F.);
#20490=ORIENTED_EDGE('',*,*,#15045,.T.);
#20491=ORIENTED_EDGE('',*,*,#15159,.F.);
#20492=ORIENTED_EDGE('',*,*,#15098,.F.);
#20493=ORIENTED_EDGE('',*,*,#15147,.F.);
#20494=ORIENTED_EDGE('',*,*,#15160,.F.);
#20495=ORIENTED_EDGE('',*,*,#15161,.T.);
#20496=ORIENTED_EDGE('',*,*,#15162,.T.);
#20497=ORIENTED_EDGE('',*,*,#15157,.T.);
#20498=ORIENTED_EDGE('',*,*,#15150,.F.);
#20499=ORIENTED_EDGE('',*,*,#15163,.T.);
#20500=ORIENTED_EDGE('',*,*,#15164,.F.);
#20501=ORIENTED_EDGE('',*,*,#15165,.T.);
#20502=ORIENTED_EDGE('',*,*,#15166,.T.);
#20503=ORIENTED_EDGE('',*,*,#15160,.T.);
#20504=ORIENTED_EDGE('',*,*,#15149,.F.);
#20505=ORIENTED_EDGE('',*,*,#15153,.F.);
#20506=ORIENTED_EDGE('',*,*,#15167,.F.);
#20507=ORIENTED_EDGE('',*,*,#15163,.F.);
#20508=ORIENTED_EDGE('',*,*,#15168,.F.);
#20509=ORIENTED_EDGE('',*,*,#15169,.F.);
#20510=ORIENTED_EDGE('',*,*,#15170,.F.);
#20511=ORIENTED_EDGE('',*,*,#15171,.F.);
#20512=ORIENTED_EDGE('',*,*,#15152,.F.);
#20513=ORIENTED_EDGE('',*,*,#15172,.T.);
#20514=ORIENTED_EDGE('',*,*,#15173,.T.);
#20515=ORIENTED_EDGE('',*,*,#15174,.T.);
#20516=ORIENTED_EDGE('',*,*,#15164,.T.);
#20517=ORIENTED_EDGE('',*,*,#15167,.T.);
#20518=ORIENTED_EDGE('',*,*,#15174,.F.);
#20519=ORIENTED_EDGE('',*,*,#15175,.T.);
#20520=ORIENTED_EDGE('',*,*,#15176,.F.);
#20521=ORIENTED_EDGE('',*,*,#15177,.F.);
#20522=ORIENTED_EDGE('',*,*,#15178,.T.);
#20523=ORIENTED_EDGE('',*,*,#15165,.F.);
#20524=ORIENTED_EDGE('',*,*,#15179,.T.);
#20525=ORIENTED_EDGE('',*,*,#15180,.T.);
#20526=ORIENTED_EDGE('',*,*,#15181,.T.);
#20527=ORIENTED_EDGE('',*,*,#15176,.T.);
#20528=ORIENTED_EDGE('',*,*,#15182,.T.);
#20529=ORIENTED_EDGE('',*,*,#15183,.T.);
#20530=ORIENTED_EDGE('',*,*,#15181,.F.);
#20531=ORIENTED_EDGE('',*,*,#15184,.T.);
#20532=ORIENTED_EDGE('',*,*,#15185,.F.);
#20533=ORIENTED_EDGE('',*,*,#15186,.T.);
#20534=ORIENTED_EDGE('',*,*,#15177,.T.);
#20535=ORIENTED_EDGE('',*,*,#15180,.F.);
#20536=ORIENTED_EDGE('',*,*,#15187,.F.);
#20537=ORIENTED_EDGE('',*,*,#15188,.F.);
#20538=ORIENTED_EDGE('',*,*,#15184,.F.);
#20539=ORIENTED_EDGE('',*,*,#15189,.F.);
#20540=ORIENTED_EDGE('',*,*,#15190,.F.);
#20541=ORIENTED_EDGE('',*,*,#15191,.F.);
#20542=ORIENTED_EDGE('',*,*,#15192,.F.);
#20543=ORIENTED_EDGE('',*,*,#15179,.F.);
#20544=ORIENTED_EDGE('',*,*,#15193,.T.);
#20545=ORIENTED_EDGE('',*,*,#15116,.T.);
#20546=ORIENTED_EDGE('',*,*,#15137,.F.);
#20547=ORIENTED_EDGE('',*,*,#15187,.T.);
#20548=ORIENTED_EDGE('',*,*,#15154,.F.);
#20549=ORIENTED_EDGE('',*,*,#15117,.T.);
#20550=ORIENTED_EDGE('',*,*,#15193,.F.);
#20551=ORIENTED_EDGE('',*,*,#15183,.F.);
#20552=ORIENTED_EDGE('',*,*,#15194,.T.);
#20553=ORIENTED_EDGE('',*,*,#15172,.F.);
#20554=ORIENTED_EDGE('',*,*,#15195,.T.);
#20555=ORIENTED_EDGE('',*,*,#15196,.T.);
#20556=ORIENTED_EDGE('',*,*,#15044,.T.);
#20557=ORIENTED_EDGE('',*,*,#15111,.F.);
#20558=ORIENTED_EDGE('',*,*,#15099,.F.);
#20559=ORIENTED_EDGE('',*,*,#15159,.T.);
#20560=ORIENTED_EDGE('',*,*,#15196,.F.);
#20561=ORIENTED_EDGE('',*,*,#15197,.T.);
#20562=ORIENTED_EDGE('',*,*,#15031,.T.);
#20563=ORIENTED_EDGE('',*,*,#15032,.F.);
#20564=ORIENTED_EDGE('',*,*,#15197,.F.);
#20565=ORIENTED_EDGE('',*,*,#15195,.F.);
#20566=ORIENTED_EDGE('',*,*,#15110,.F.);
#20567=ORIENTED_EDGE('',*,*,#15071,.F.);
#20568=ORIENTED_EDGE('',*,*,#15060,.F.);
#20569=ORIENTED_EDGE('',*,*,#15198,.F.);
#20570=ORIENTED_EDGE('',*,*,#15199,.F.);
#20571=ORIENTED_EDGE('',*,*,#15200,.F.);
#20572=ORIENTED_EDGE('',*,*,#15201,.F.);
#20573=ORIENTED_EDGE('',*,*,#15202,.F.);
#20574=ORIENTED_EDGE('',*,*,#15203,.F.);
#20575=ORIENTED_EDGE('',*,*,#15204,.F.);
#20576=ORIENTED_EDGE('',*,*,#15161,.F.);
#20577=ORIENTED_EDGE('',*,*,#15166,.F.);
#20578=ORIENTED_EDGE('',*,*,#15178,.F.);
#20579=ORIENTED_EDGE('',*,*,#15186,.F.);
#20580=ORIENTED_EDGE('',*,*,#15205,.F.);
#20581=ORIENTED_EDGE('',*,*,#15134,.F.);
#20582=ORIENTED_EDGE('',*,*,#15026,.F.);
#20583=ORIENTED_EDGE('',*,*,#15205,.T.);
#20584=ORIENTED_EDGE('',*,*,#15185,.T.);
#20585=ORIENTED_EDGE('',*,*,#15206,.T.);
#20586=ORIENTED_EDGE('',*,*,#15135,.F.);
#20587=ORIENTED_EDGE('',*,*,#15136,.F.);
#20588=ORIENTED_EDGE('',*,*,#15133,.F.);
#20589=ORIENTED_EDGE('',*,*,#15206,.F.);
#20590=ORIENTED_EDGE('',*,*,#15188,.T.);
#20591=ORIENTED_EDGE('',*,*,#15207,.F.);
#20592=ORIENTED_EDGE('',*,*,#15208,.F.);
#20593=ORIENTED_EDGE('',*,*,#15209,.F.);
#20594=ORIENTED_EDGE('',*,*,#15203,.T.);
#20595=ORIENTED_EDGE('',*,*,#15208,.T.);
#20596=ORIENTED_EDGE('',*,*,#15210,.T.);
#20597=ORIENTED_EDGE('',*,*,#15211,.T.);
#20598=ORIENTED_EDGE('',*,*,#15212,.T.);
#20599=ORIENTED_EDGE('',*,*,#15213,.T.);
#20600=ORIENTED_EDGE('',*,*,#15209,.T.);
#20601=ORIENTED_EDGE('',*,*,#15202,.T.);
#20602=ORIENTED_EDGE('',*,*,#15214,.T.);
#20603=ORIENTED_EDGE('',*,*,#15139,.F.);
#20604=ORIENTED_EDGE('',*,*,#15215,.T.);
#20605=ORIENTED_EDGE('',*,*,#15207,.T.);
#20606=ORIENTED_EDGE('',*,*,#15216,.T.);
#20607=ORIENTED_EDGE('',*,*,#15217,.T.);
#20608=ORIENTED_EDGE('',*,*,#15204,.T.);
#20609=ORIENTED_EDGE('',*,*,#15211,.F.);
#20610=ORIENTED_EDGE('',*,*,#15218,.T.);
#20611=ORIENTED_EDGE('',*,*,#15162,.F.);
#20612=ORIENTED_EDGE('',*,*,#15140,.F.);
#20613=ORIENTED_EDGE('',*,*,#15217,.F.);
#20614=ORIENTED_EDGE('',*,*,#15219,.T.);
#20615=ORIENTED_EDGE('',*,*,#15220,.T.);
#20616=ORIENTED_EDGE('',*,*,#15221,.T.);
#20617=ORIENTED_EDGE('',*,*,#15122,.T.);
#20618=ORIENTED_EDGE('',*,*,#15087,.F.);
#20619=ORIENTED_EDGE('',*,*,#15158,.F.);
#20620=ORIENTED_EDGE('',*,*,#15218,.F.);
#20621=ORIENTED_EDGE('',*,*,#15222,.F.);
#20622=ORIENTED_EDGE('',*,*,#15093,.F.);
#20623=ORIENTED_EDGE('',*,*,#15112,.F.);
#20624=ORIENTED_EDGE('',*,*,#15043,.T.);
#20625=ORIENTED_EDGE('',*,*,#15039,.F.);
#20626=ORIENTED_EDGE('',*,*,#15089,.T.);
#20627=ORIENTED_EDGE('',*,*,#15084,.F.);
#20628=ORIENTED_EDGE('',*,*,#15222,.T.);
#20629=ORIENTED_EDGE('',*,*,#15210,.F.);
#20630=ORIENTED_EDGE('',*,*,#15215,.F.);
#20631=ORIENTED_EDGE('',*,*,#15138,.F.);
#20632=ORIENTED_EDGE('',*,*,#15155,.T.);
#20633=ORIENTED_EDGE('',*,*,#15035,.F.);
#20634=ORIENTED_EDGE('',*,*,#15037,.T.);
#20635=ORIENTED_EDGE('',*,*,#15011,.F.);
#20636=ORIENTED_EDGE('',*,*,#15015,.T.);
#20637=ORIENTED_EDGE('',*,*,#15109,.F.);
#20638=ORIENTED_EDGE('',*,*,#15221,.F.);
#20639=ORIENTED_EDGE('',*,*,#15223,.F.);
#20640=ORIENTED_EDGE('',*,*,#15224,.T.);
#20641=ORIENTED_EDGE('',*,*,#15225,.F.);
#20642=ORIENTED_EDGE('',*,*,#15226,.F.);
#20643=ORIENTED_EDGE('',*,*,#15123,.T.);
#20644=ORIENTED_EDGE('',*,*,#15083,.T.);
#20645=ORIENTED_EDGE('',*,*,#15227,.T.);
#20646=ORIENTED_EDGE('',*,*,#15199,.T.);
#20647=ORIENTED_EDGE('',*,*,#15228,.T.);
#20648=ORIENTED_EDGE('',*,*,#15048,.F.);
#20649=ORIENTED_EDGE('',*,*,#15081,.T.);
#20650=ORIENTED_EDGE('',*,*,#15228,.F.);
#20651=ORIENTED_EDGE('',*,*,#15198,.T.);
#20652=ORIENTED_EDGE('',*,*,#15059,.T.);
#20653=ORIENTED_EDGE('',*,*,#15229,.T.);
#20654=ORIENTED_EDGE('',*,*,#15230,.T.);
#20655=ORIENTED_EDGE('',*,*,#15078,.F.);
#20656=ORIENTED_EDGE('',*,*,#15124,.T.);
#20657=ORIENTED_EDGE('',*,*,#15226,.T.);
#20658=ORIENTED_EDGE('',*,*,#15230,.F.);
#20659=ORIENTED_EDGE('',*,*,#15231,.F.);
#20660=ORIENTED_EDGE('',*,*,#15232,.F.);
#20661=ORIENTED_EDGE('',*,*,#15082,.T.);
#20662=ORIENTED_EDGE('',*,*,#15233,.F.);
#20663=ORIENTED_EDGE('',*,*,#15234,.F.);
#20664=ORIENTED_EDGE('',*,*,#15235,.F.);
#20665=ORIENTED_EDGE('',*,*,#15236,.F.);
#20666=ORIENTED_EDGE('',*,*,#15229,.F.);
#20667=ORIENTED_EDGE('',*,*,#15225,.T.);
#20668=ORIENTED_EDGE('',*,*,#15237,.T.);
#20669=ORIENTED_EDGE('',*,*,#15238,.T.);
#20670=ORIENTED_EDGE('',*,*,#15239,.F.);
#20671=ORIENTED_EDGE('',*,*,#15231,.T.);
#20672=ORIENTED_EDGE('',*,*,#15240,.T.);
#20673=ORIENTED_EDGE('',*,*,#15200,.T.);
#20674=ORIENTED_EDGE('',*,*,#15227,.F.);
#20675=ORIENTED_EDGE('',*,*,#15232,.T.);
#20676=ORIENTED_EDGE('',*,*,#15239,.T.);
#20677=ORIENTED_EDGE('',*,*,#15214,.F.);
#20678=ORIENTED_EDGE('',*,*,#15201,.T.);
#20679=ORIENTED_EDGE('',*,*,#15240,.F.);
#20680=ORIENTED_EDGE('',*,*,#15238,.F.);
#20681=ORIENTED_EDGE('',*,*,#15241,.T.);
#20682=ORIENTED_EDGE('',*,*,#15242,.F.);
#20683=ORIENTED_EDGE('',*,*,#15212,.F.);
#20684=ORIENTED_EDGE('',*,*,#15242,.T.);
#20685=ORIENTED_EDGE('',*,*,#15243,.T.);
#20686=ORIENTED_EDGE('',*,*,#15223,.T.);
#20687=ORIENTED_EDGE('',*,*,#15220,.F.);
#20688=ORIENTED_EDGE('',*,*,#15244,.T.);
#20689=ORIENTED_EDGE('',*,*,#15213,.F.);
#20690=ORIENTED_EDGE('',*,*,#15244,.F.);
#20691=ORIENTED_EDGE('',*,*,#15219,.F.);
#20692=ORIENTED_EDGE('',*,*,#15216,.F.);
#20693=ORIENTED_EDGE('',*,*,#15245,.F.);
#20694=ORIENTED_EDGE('',*,*,#15246,.F.);
#20695=ORIENTED_EDGE('',*,*,#15247,.F.);
#20696=ORIENTED_EDGE('',*,*,#15248,.F.);
#20697=ORIENTED_EDGE('',*,*,#15249,.T.);
#20698=ORIENTED_EDGE('',*,*,#15189,.T.);
#20699=ORIENTED_EDGE('',*,*,#15250,.T.);
#20700=ORIENTED_EDGE('',*,*,#15251,.T.);
#20701=ORIENTED_EDGE('',*,*,#15252,.T.);
#20702=ORIENTED_EDGE('',*,*,#15190,.T.);
#20703=ORIENTED_EDGE('',*,*,#15249,.F.);
#20704=ORIENTED_EDGE('',*,*,#15253,.T.);
#20705=ORIENTED_EDGE('',*,*,#15254,.T.);
#20706=ORIENTED_EDGE('',*,*,#15191,.T.);
#20707=ORIENTED_EDGE('',*,*,#15252,.F.);
#20708=ORIENTED_EDGE('',*,*,#15255,.T.);
#20709=ORIENTED_EDGE('',*,*,#15250,.F.);
#20710=ORIENTED_EDGE('',*,*,#15192,.T.);
#20711=ORIENTED_EDGE('',*,*,#15254,.F.);
#20712=ORIENTED_EDGE('',*,*,#15256,.T.);
#20713=ORIENTED_EDGE('',*,*,#15253,.F.);
#20714=ORIENTED_EDGE('',*,*,#15257,.F.);
#20715=ORIENTED_EDGE('',*,*,#15258,.F.);
#20716=ORIENTED_EDGE('',*,*,#15259,.T.);
#20717=ORIENTED_EDGE('',*,*,#15251,.F.);
#20718=ORIENTED_EDGE('',*,*,#15260,.F.);
#20719=ORIENTED_EDGE('',*,*,#15261,.F.);
#20720=ORIENTED_EDGE('',*,*,#15257,.T.);
#20721=ORIENTED_EDGE('',*,*,#15262,.T.);
#20722=ORIENTED_EDGE('',*,*,#15168,.T.);
#20723=ORIENTED_EDGE('',*,*,#15263,.T.);
#20724=ORIENTED_EDGE('',*,*,#15261,.T.);
#20725=ORIENTED_EDGE('',*,*,#15264,.T.);
#20726=ORIENTED_EDGE('',*,*,#15169,.T.);
#20727=ORIENTED_EDGE('',*,*,#15262,.F.);
#20728=ORIENTED_EDGE('',*,*,#15265,.T.);
#20729=ORIENTED_EDGE('',*,*,#15266,.T.);
#20730=ORIENTED_EDGE('',*,*,#15170,.T.);
#20731=ORIENTED_EDGE('',*,*,#15264,.F.);
#20732=ORIENTED_EDGE('',*,*,#15267,.T.);
#20733=ORIENTED_EDGE('',*,*,#15263,.F.);
#20734=ORIENTED_EDGE('',*,*,#15171,.T.);
#20735=ORIENTED_EDGE('',*,*,#15266,.F.);
#20736=ORIENTED_EDGE('',*,*,#15258,.T.);
#20737=ORIENTED_EDGE('',*,*,#15256,.F.);
#20738=ORIENTED_EDGE('',*,*,#15268,.F.);
#20739=ORIENTED_EDGE('',*,*,#15265,.F.);
#20740=ORIENTED_EDGE('',*,*,#15260,.T.);
#20741=ORIENTED_EDGE('',*,*,#15269,.T.);
#20742=ORIENTED_EDGE('',*,*,#15233,.T.);
#20743=ORIENTED_EDGE('',*,*,#15270,.T.);
#20744=ORIENTED_EDGE('',*,*,#15271,.T.);
#20745=ORIENTED_EDGE('',*,*,#15272,.T.);
#20746=ORIENTED_EDGE('',*,*,#15234,.T.);
#20747=ORIENTED_EDGE('',*,*,#15269,.F.);
#20748=ORIENTED_EDGE('',*,*,#15273,.T.);
#20749=ORIENTED_EDGE('',*,*,#15274,.T.);
#20750=ORIENTED_EDGE('',*,*,#15235,.T.);
#20751=ORIENTED_EDGE('',*,*,#15272,.F.);
#20752=ORIENTED_EDGE('',*,*,#15275,.T.);
#20753=ORIENTED_EDGE('',*,*,#15270,.F.);
#20754=ORIENTED_EDGE('',*,*,#15236,.T.);
#20755=ORIENTED_EDGE('',*,*,#15274,.F.);
#20756=ORIENTED_EDGE('',*,*,#15276,.T.);
#20757=ORIENTED_EDGE('',*,*,#15273,.F.);
#20758=ORIENTED_EDGE('',*,*,#15277,.F.);
#20759=ORIENTED_EDGE('',*,*,#15278,.F.);
#20760=ORIENTED_EDGE('',*,*,#15279,.T.);
#20761=ORIENTED_EDGE('',*,*,#15271,.F.);
#20762=ORIENTED_EDGE('',*,*,#15280,.F.);
#20763=ORIENTED_EDGE('',*,*,#15281,.F.);
#20764=ORIENTED_EDGE('',*,*,#15277,.T.);
#20765=ORIENTED_EDGE('',*,*,#15282,.T.);
#20766=ORIENTED_EDGE('',*,*,#15245,.T.);
#20767=ORIENTED_EDGE('',*,*,#15283,.T.);
#20768=ORIENTED_EDGE('',*,*,#15281,.T.);
#20769=ORIENTED_EDGE('',*,*,#15284,.T.);
#20770=ORIENTED_EDGE('',*,*,#15246,.T.);
#20771=ORIENTED_EDGE('',*,*,#15282,.F.);
#20772=ORIENTED_EDGE('',*,*,#15285,.T.);
#20773=ORIENTED_EDGE('',*,*,#15286,.T.);
#20774=ORIENTED_EDGE('',*,*,#15247,.T.);
#20775=ORIENTED_EDGE('',*,*,#15284,.F.);
#20776=ORIENTED_EDGE('',*,*,#15287,.T.);
#20777=ORIENTED_EDGE('',*,*,#15283,.F.);
#20778=ORIENTED_EDGE('',*,*,#15248,.T.);
#20779=ORIENTED_EDGE('',*,*,#15286,.F.);
#20780=ORIENTED_EDGE('',*,*,#15278,.T.);
#20781=ORIENTED_EDGE('',*,*,#15276,.F.);
#20782=ORIENTED_EDGE('',*,*,#15288,.F.);
#20783=ORIENTED_EDGE('',*,*,#15285,.F.);
#20784=ORIENTED_EDGE('',*,*,#15280,.T.);
#20785=ORIENTED_EDGE('',*,*,#15275,.F.);
#20786=ORIENTED_EDGE('',*,*,#15279,.F.);
#20787=ORIENTED_EDGE('',*,*,#15287,.F.);
#20788=ORIENTED_EDGE('',*,*,#15288,.T.);
#20789=ORIENTED_EDGE('',*,*,#15255,.F.);
#20790=ORIENTED_EDGE('',*,*,#15259,.F.);
#20791=ORIENTED_EDGE('',*,*,#15267,.F.);
#20792=ORIENTED_EDGE('',*,*,#15268,.T.);
#20793=ORIENTED_EDGE('',*,*,#15243,.F.);
#20794=ORIENTED_EDGE('',*,*,#15241,.F.);
#20795=ORIENTED_EDGE('',*,*,#15237,.F.);
#20796=ORIENTED_EDGE('',*,*,#15224,.F.);
#20797=ORIENTED_EDGE('',*,*,#15021,.F.);
#20798=ORIENTED_EDGE('',*,*,#15024,.T.);
#20799=ORIENTED_EDGE('',*,*,#15125,.F.);
#20800=ORIENTED_EDGE('',*,*,#15131,.F.);
#20801=ORIENTED_EDGE('',*,*,#15113,.T.);
#20802=ORIENTED_EDGE('',*,*,#15100,.F.);
#20803=ORIENTED_EDGE('',*,*,#15173,.F.);
#20804=ORIENTED_EDGE('',*,*,#15194,.F.);
#20805=ORIENTED_EDGE('',*,*,#15182,.F.);
#20806=ORIENTED_EDGE('',*,*,#15175,.F.);
#20807=ORIENTED_EDGE('',*,*,#15017,.F.);
#20808=ORIENTED_EDGE('',*,*,#15102,.F.);
#20809=ORIENTED_EDGE('',*,*,#15097,.F.);
#20810=ORIENTED_EDGE('',*,*,#15029,.F.);
#26279=PLANE('',#29182);
#26280=PLANE('',#29183);
#26281=PLANE('',#29184);
#26282=PLANE('',#29185);
#26283=PLANE('',#29186);
#26284=PLANE('',#29187);
#26285=PLANE('',#29188);
#26286=PLANE('',#29189);
#26287=PLANE('',#29190);
#26288=PLANE('',#29191);
#26289=PLANE('',#29192);
#26290=PLANE('',#29193);
#26291=PLANE('',#29194);
#26292=PLANE('',#29195);
#26293=PLANE('',#29196);
#26294=PLANE('',#29197);
#26295=PLANE('',#29198);
#26296=PLANE('',#29199);
#26297=PLANE('',#29200);
#26298=PLANE('',#29201);
#26299=PLANE('',#29202);
#26300=PLANE('',#29203);
#26301=PLANE('',#29204);
#26302=PLANE('',#29205);
#26303=PLANE('',#29206);
#26304=PLANE('',#29207);
#26305=PLANE('',#29208);
#26306=PLANE('',#29209);
#26307=PLANE('',#29210);
#26308=PLANE('',#29211);
#26309=PLANE('',#29212);
#26310=PLANE('',#29213);
#26311=PLANE('',#29214);
#26312=PLANE('',#29215);
#26313=PLANE('',#29216);
#26314=PLANE('',#29217);
#26315=PLANE('',#29218);
#26316=PLANE('',#29219);
#26317=PLANE('',#29220);
#26318=PLANE('',#29221);
#26319=PLANE('',#29222);
#26320=PLANE('',#29223);
#26321=PLANE('',#29224);
#26322=PLANE('',#29225);
#26323=PLANE('',#29226);
#26324=PLANE('',#29227);
#26325=PLANE('',#29228);
#26326=PLANE('',#29229);
#26327=PLANE('',#29230);
#26328=PLANE('',#29231);
#26329=PLANE('',#29234);
#26330=PLANE('',#29235);
#26331=PLANE('',#29236);
#26332=PLANE('',#29237);
#26333=PLANE('',#29238);
#26334=PLANE('',#29241);
#26335=PLANE('',#29242);
#26336=PLANE('',#29243);
#26337=PLANE('',#29244);
#26338=PLANE('',#29245);
#26339=PLANE('',#29246);
#26340=PLANE('',#29247);
#26341=PLANE('',#29248);
#26342=PLANE('',#29249);
#26343=PLANE('',#29250);
#26344=PLANE('',#29251);
#26345=PLANE('',#29252);
#26346=PLANE('',#29253);
#26347=PLANE('',#29254);
#26348=PLANE('',#29255);
#26349=PLANE('',#29256);
#26350=PLANE('',#29257);
#26351=PLANE('',#29258);
#26352=PLANE('',#29259);
#26353=PLANE('',#29260);
#26354=PLANE('',#29263);
#26355=PLANE('',#29264);
#26356=PLANE('',#29265);
#26357=PLANE('',#29266);
#26358=PLANE('',#29267);
#26359=PLANE('',#29270);
#26360=PLANE('',#29273);
#26361=PLANE('',#29278);
#26362=PLANE('',#29279);
#26363=PLANE('',#29282);
#26364=PLANE('',#29285);
#26365=PLANE('',#29288);
#26366=PLANE('',#29293);
#26367=PLANE('',#29294);
#26368=PLANE('',#29297);
#26369=PLANE('',#29300);
#26370=PLANE('',#29301);
#26371=PLANE('',#29302);
#26372=PLANE('',#29303);
#26373=PLANE('',#29304);
#26374=PLANE('',#29305);
#27306=ADVANCED_FACE('',(#3398),#26279,.T.);
#27307=ADVANCED_FACE('',(#3399),#26280,.F.);
#27308=ADVANCED_FACE('',(#3400),#26281,.T.);
#27309=ADVANCED_FACE('',(#3401),#26282,.T.);
#27310=ADVANCED_FACE('',(#3402),#26283,.T.);
#27311=ADVANCED_FACE('',(#3403),#26284,.T.);
#27312=ADVANCED_FACE('',(#3404),#26285,.T.);
#27313=ADVANCED_FACE('',(#3405),#26286,.T.);
#27314=ADVANCED_FACE('',(#3406),#26287,.T.);
#27315=ADVANCED_FACE('',(#3407),#26288,.F.);
#27316=ADVANCED_FACE('',(#3408),#26289,.T.);
#27317=ADVANCED_FACE('',(#3409),#26290,.T.);
#27318=ADVANCED_FACE('',(#3410),#26291,.T.);
#27319=ADVANCED_FACE('',(#3411),#26292,.T.);
#27320=ADVANCED_FACE('',(#3412),#26293,.T.);
#27321=ADVANCED_FACE('',(#3413),#26294,.T.);
#27322=ADVANCED_FACE('',(#3414),#26295,.T.);
#27323=ADVANCED_FACE('',(#3415),#26296,.T.);
#27324=ADVANCED_FACE('',(#3416),#26297,.T.);
#27325=ADVANCED_FACE('',(#3417),#26298,.T.);
#27326=ADVANCED_FACE('',(#3418),#26299,.T.);
#27327=ADVANCED_FACE('',(#3419),#26300,.T.);
#27328=ADVANCED_FACE('',(#3420),#26301,.T.);
#27329=ADVANCED_FACE('',(#3421),#26302,.T.);
#27330=ADVANCED_FACE('',(#3422),#26303,.T.);
#27331=ADVANCED_FACE('',(#3423),#26304,.T.);
#27332=ADVANCED_FACE('',(#3424),#26305,.T.);
#27333=ADVANCED_FACE('',(#3425),#26306,.T.);
#27334=ADVANCED_FACE('',(#3426),#26307,.T.);
#27335=ADVANCED_FACE('',(#3427),#26308,.T.);
#27336=ADVANCED_FACE('',(#3428),#26309,.T.);
#27337=ADVANCED_FACE('',(#3429),#26310,.T.);
#27338=ADVANCED_FACE('',(#3430),#26311,.T.);
#27339=ADVANCED_FACE('',(#3431),#26312,.T.);
#27340=ADVANCED_FACE('',(#3432),#26313,.T.);
#27341=ADVANCED_FACE('',(#3433),#26314,.T.);
#27342=ADVANCED_FACE('',(#3434),#26315,.T.);
#27343=ADVANCED_FACE('',(#3435),#26316,.T.);
#27344=ADVANCED_FACE('',(#3436),#26317,.T.);
#27345=ADVANCED_FACE('',(#3437),#26318,.T.);
#27346=ADVANCED_FACE('',(#3438),#26319,.T.);
#27347=ADVANCED_FACE('',(#3439),#26320,.T.);
#27348=ADVANCED_FACE('',(#3440),#26321,.T.);
#27349=ADVANCED_FACE('',(#3441),#26322,.T.);
#27350=ADVANCED_FACE('',(#3442),#26323,.T.);
#27351=ADVANCED_FACE('',(#3443),#26324,.T.);
#27352=ADVANCED_FACE('',(#3444),#26325,.T.);
#27353=ADVANCED_FACE('',(#3445),#26326,.T.);
#27354=ADVANCED_FACE('',(#3446),#26327,.T.);
#27355=ADVANCED_FACE('',(#3447,#1910),#26328,.T.);
#27356=ADVANCED_FACE('',(#3448),#26329,.T.);
#27357=ADVANCED_FACE('',(#3449),#26330,.T.);
#27358=ADVANCED_FACE('',(#3450),#26331,.T.);
#27359=ADVANCED_FACE('',(#3451),#26332,.T.);
#27360=ADVANCED_FACE('',(#3452,#1911),#26333,.T.);
#27361=ADVANCED_FACE('',(#3453),#26334,.T.);
#27362=ADVANCED_FACE('',(#3454),#26335,.T.);
#27363=ADVANCED_FACE('',(#3455),#26336,.T.);
#27364=ADVANCED_FACE('',(#3456),#26337,.T.);
#27365=ADVANCED_FACE('',(#3457),#26338,.F.);
#27366=ADVANCED_FACE('',(#3458),#26339,.T.);
#27367=ADVANCED_FACE('',(#3459),#26340,.T.);
#27368=ADVANCED_FACE('',(#3460),#26341,.T.);
#27369=ADVANCED_FACE('',(#3461),#26342,.T.);
#27370=ADVANCED_FACE('',(#3462),#26343,.T.);
#27371=ADVANCED_FACE('',(#3463),#26344,.T.);
#27372=ADVANCED_FACE('',(#3464),#26345,.T.);
#27373=ADVANCED_FACE('',(#3465),#26346,.T.);
#27374=ADVANCED_FACE('',(#3466),#26347,.T.);
#27375=ADVANCED_FACE('',(#3467),#26348,.T.);
#27376=ADVANCED_FACE('',(#3468),#26349,.T.);
#27377=ADVANCED_FACE('',(#3469),#26350,.T.);
#27378=ADVANCED_FACE('',(#3470),#26351,.T.);
#27379=ADVANCED_FACE('',(#3471),#26352,.T.);
#27380=ADVANCED_FACE('',(#3472,#1912),#26353,.T.);
#27381=ADVANCED_FACE('',(#3473),#26354,.T.);
#27382=ADVANCED_FACE('',(#3474),#26355,.T.);
#27383=ADVANCED_FACE('',(#3475),#26356,.T.);
#27384=ADVANCED_FACE('',(#3476),#26357,.T.);
#27385=ADVANCED_FACE('',(#3477,#1913),#26358,.T.);
#27386=ADVANCED_FACE('',(#3478),#26359,.T.);
#27387=ADVANCED_FACE('',(#3479),#2807,.F.);
#27388=ADVANCED_FACE('',(#3480),#26360,.T.);
#27389=ADVANCED_FACE('',(#3481),#2808,.F.);
#27390=ADVANCED_FACE('',(#3482),#1569,.F.);
#27391=ADVANCED_FACE('',(#3483),#26361,.F.);
#27392=ADVANCED_FACE('',(#3484),#26362,.T.);
#27393=ADVANCED_FACE('',(#3485),#2809,.F.);
#27394=ADVANCED_FACE('',(#3486),#26363,.T.);
#27395=ADVANCED_FACE('',(#3487),#2810,.F.);
#27396=ADVANCED_FACE('',(#3488),#1570,.F.);
#27397=ADVANCED_FACE('',(#3489),#26364,.T.);
#27398=ADVANCED_FACE('',(#3490),#2811,.F.);
#27399=ADVANCED_FACE('',(#3491),#26365,.T.);
#27400=ADVANCED_FACE('',(#3492),#2812,.F.);
#27401=ADVANCED_FACE('',(#3493),#1571,.F.);
#27402=ADVANCED_FACE('',(#3494),#26366,.F.);
#27403=ADVANCED_FACE('',(#3495),#26367,.T.);
#27404=ADVANCED_FACE('',(#3496),#2813,.F.);
#27405=ADVANCED_FACE('',(#3497),#26368,.T.);
#27406=ADVANCED_FACE('',(#3498),#2814,.F.);
#27407=ADVANCED_FACE('',(#3499),#1572,.F.);
#27408=ADVANCED_FACE('',(#3500),#26369,.F.);
#27409=ADVANCED_FACE('',(#3501),#26370,.F.);
#27410=ADVANCED_FACE('',(#3502),#26371,.T.);
#27411=ADVANCED_FACE('',(#3503),#26372,.T.);
#27412=ADVANCED_FACE('',(#3504),#26373,.T.);
#27413=ADVANCED_FACE('',(#3505),#26374,.T.);
#28461=CLOSED_SHELL('',(#27306,#27307,#27308,#27309,#27310,#27311,#27312,
#27313,#27314,#27315,#27316,#27317,#27318,#27319,#27320,#27321,#27322,#27323,
#27324,#27325,#27326,#27327,#27328,#27329,#27330,#27331,#27332,#27333,#27334,
#27335,#27336,#27337,#27338,#27339,#27340,#27341,#27342,#27343,#27344,#27345,
#27346,#27347,#27348,#27349,#27350,#27351,#27352,#27353,#27354,#27355,#27356,
#27357,#27358,#27359,#27360,#27361,#27362,#27363,#27364,#27365,#27366,#27367,
#27368,#27369,#27370,#27371,#27372,#27373,#27374,#27375,#27376,#27377,#27378,
#27379,#27380,#27381,#27382,#27383,#27384,#27385,#27386,#27387,#27388,#27389,
#27390,#27391,#27392,#27393,#27394,#27395,#27396,#27397,#27398,#27399,#27400,
#27401,#27402,#27403,#27404,#27405,#27406,#27407,#27408,#27409,#27410,#27411,
#27412,#27413));
#29181=AXIS2_PLACEMENT_3D('',#42803,#32604,#32605);
#29182=AXIS2_PLACEMENT_3D('',#42804,#32606,#32607);
#29183=AXIS2_PLACEMENT_3D('',#42813,#32612,#32613);
#29184=AXIS2_PLACEMENT_3D('',#42819,#32617,#32618);
#29185=AXIS2_PLACEMENT_3D('',#42832,#32625,#32626);
#29186=AXIS2_PLACEMENT_3D('',#42838,#32630,#32631);
#29187=AXIS2_PLACEMENT_3D('',#42846,#32636,#32637);
#29188=AXIS2_PLACEMENT_3D('',#42854,#32642,#32643);
#29189=AXIS2_PLACEMENT_3D('',#42863,#32648,#32649);
#29190=AXIS2_PLACEMENT_3D('',#42866,#32652,#32653);
#29191=AXIS2_PLACEMENT_3D('',#42875,#32658,#32659);
#29192=AXIS2_PLACEMENT_3D('',#42881,#32663,#32664);
#29193=AXIS2_PLACEMENT_3D('',#42894,#32671,#32672);
#29194=AXIS2_PLACEMENT_3D('',#42904,#32678,#32679);
#29195=AXIS2_PLACEMENT_3D('',#42908,#32682,#32683);
#29196=AXIS2_PLACEMENT_3D('',#42916,#32688,#32689);
#29197=AXIS2_PLACEMENT_3D('',#42922,#32693,#32694);
#29198=AXIS2_PLACEMENT_3D('',#42928,#32698,#32699);
#29199=AXIS2_PLACEMENT_3D('',#42932,#32702,#32703);
#29200=AXIS2_PLACEMENT_3D('',#42938,#32707,#32708);
#29201=AXIS2_PLACEMENT_3D('',#42944,#32712,#32713);
#29202=AXIS2_PLACEMENT_3D('',#42950,#32717,#32718);
#29203=AXIS2_PLACEMENT_3D('',#42954,#32721,#32722);
#29204=AXIS2_PLACEMENT_3D('',#42958,#32725,#32726);
#29205=AXIS2_PLACEMENT_3D('',#42967,#32731,#32732);
#29206=AXIS2_PLACEMENT_3D('',#42970,#32735,#32736);
#29207=AXIS2_PLACEMENT_3D('',#42974,#32739,#32740);
#29208=AXIS2_PLACEMENT_3D('',#42978,#32743,#32744);
#29209=AXIS2_PLACEMENT_3D('',#42985,#32748,#32749);
#29210=AXIS2_PLACEMENT_3D('',#42990,#32753,#32754);
#29211=AXIS2_PLACEMENT_3D('',#42995,#32758,#32759);
#29212=AXIS2_PLACEMENT_3D('',#43000,#32763,#32764);
#29213=AXIS2_PLACEMENT_3D('',#43004,#32767,#32768);
#29214=AXIS2_PLACEMENT_3D('',#43007,#32771,#32772);
#29215=AXIS2_PLACEMENT_3D('',#43012,#32776,#32777);
#29216=AXIS2_PLACEMENT_3D('',#43036,#32790,#32791);
#29217=AXIS2_PLACEMENT_3D('',#43044,#32796,#32797);
#29218=AXIS2_PLACEMENT_3D('',#43049,#32801,#32802);
#29219=AXIS2_PLACEMENT_3D('',#43053,#32805,#32806);
#29220=AXIS2_PLACEMENT_3D('',#43057,#32809,#32810);
#29221=AXIS2_PLACEMENT_3D('',#43061,#32813,#32814);
#29222=AXIS2_PLACEMENT_3D('',#43069,#32819,#32820);
#29223=AXIS2_PLACEMENT_3D('',#43073,#32823,#32824);
#29224=AXIS2_PLACEMENT_3D('',#43079,#32828,#32829);
#29225=AXIS2_PLACEMENT_3D('',#43087,#32834,#32835);
#29226=AXIS2_PLACEMENT_3D('',#43089,#32837,#32838);
#29227=AXIS2_PLACEMENT_3D('',#43095,#32842,#32843);
#29228=AXIS2_PLACEMENT_3D('',#43098,#32846,#32847);
#29229=AXIS2_PLACEMENT_3D('',#43103,#32851,#32852);
#29230=AXIS2_PLACEMENT_3D('',#43109,#32856,#32857);
#29231=AXIS2_PLACEMENT_3D('',#43117,#32862,#32863);
#29232=AXIS2_PLACEMENT_3D('',#43123,#32866,#32867);
#29233=AXIS2_PLACEMENT_3D('',#43126,#32869,#32870);
#29234=AXIS2_PLACEMENT_3D('',#43127,#32871,#32872);
#29235=AXIS2_PLACEMENT_3D('',#43133,#32876,#32877);
#29236=AXIS2_PLACEMENT_3D('',#43141,#32882,#32883);
#29237=AXIS2_PLACEMENT_3D('',#43151,#32889,#32890);
#29238=AXIS2_PLACEMENT_3D('',#43157,#32894,#32895);
#29239=AXIS2_PLACEMENT_3D('',#43164,#32899,#32900);
#29240=AXIS2_PLACEMENT_3D('',#43167,#32902,#32903);
#29241=AXIS2_PLACEMENT_3D('',#43168,#32904,#32905);
#29242=AXIS2_PLACEMENT_3D('',#43170,#32907,#32908);
#29243=AXIS2_PLACEMENT_3D('',#43172,#32910,#32911);
#29244=AXIS2_PLACEMENT_3D('',#43176,#32914,#32915);
#29245=AXIS2_PLACEMENT_3D('',#43178,#32917,#32918);
#29246=AXIS2_PLACEMENT_3D('',#43193,#32927,#32928);
#29247=AXIS2_PLACEMENT_3D('',#43195,#32930,#32931);
#29248=AXIS2_PLACEMENT_3D('',#43196,#32932,#32933);
#29249=AXIS2_PLACEMENT_3D('',#43202,#32937,#32938);
#29250=AXIS2_PLACEMENT_3D('',#43206,#32941,#32942);
#29251=AXIS2_PLACEMENT_3D('',#43212,#32946,#32947);
#29252=AXIS2_PLACEMENT_3D('',#43217,#32951,#32952);
#29253=AXIS2_PLACEMENT_3D('',#43219,#32954,#32955);
#29254=AXIS2_PLACEMENT_3D('',#43225,#32959,#32960);
#29255=AXIS2_PLACEMENT_3D('',#43227,#32962,#32963);
#29256=AXIS2_PLACEMENT_3D('',#43228,#32964,#32965);
#29257=AXIS2_PLACEMENT_3D('',#43236,#32970,#32971);
#29258=AXIS2_PLACEMENT_3D('',#43239,#32974,#32975);
#29259=AXIS2_PLACEMENT_3D('',#43240,#32976,#32977);
#29260=AXIS2_PLACEMENT_3D('',#43244,#32980,#32981);
#29261=AXIS2_PLACEMENT_3D('',#43252,#32985,#32986);
#29262=AXIS2_PLACEMENT_3D('',#43255,#32988,#32989);
#29263=AXIS2_PLACEMENT_3D('',#43256,#32990,#32991);
#29264=AXIS2_PLACEMENT_3D('',#43262,#32995,#32996);
#29265=AXIS2_PLACEMENT_3D('',#43264,#32998,#32999);
#29266=AXIS2_PLACEMENT_3D('',#43268,#33002,#33003);
#29267=AXIS2_PLACEMENT_3D('',#43271,#33006,#33007);
#29268=AXIS2_PLACEMENT_3D('',#43276,#33009,#33010);
#29269=AXIS2_PLACEMENT_3D('',#43279,#33012,#33013);
#29270=AXIS2_PLACEMENT_3D('',#43280,#33014,#33015);
#29271=AXIS2_PLACEMENT_3D('',#43286,#33019,#33020);
#29272=AXIS2_PLACEMENT_3D('',#43289,#33022,#33023);
#29273=AXIS2_PLACEMENT_3D('',#43290,#33024,#33025);
#29274=AXIS2_PLACEMENT_3D('',#43294,#33028,#33029);
#29275=AXIS2_PLACEMENT_3D('',#43295,#33030,#33031);
#29276=AXIS2_PLACEMENT_3D('',#43296,#33032,#33033);
#29277=AXIS2_PLACEMENT_3D('',#43300,#33035,#33036);
#29278=AXIS2_PLACEMENT_3D('',#43302,#33038,#33039);
#29279=AXIS2_PLACEMENT_3D('',#43306,#33042,#33043);
#29280=AXIS2_PLACEMENT_3D('',#43309,#33046,#33047);
#29281=AXIS2_PLACEMENT_3D('',#43312,#33049,#33050);
#29282=AXIS2_PLACEMENT_3D('',#43313,#33051,#33052);
#29283=AXIS2_PLACEMENT_3D('',#43316,#33055,#33056);
#29284=AXIS2_PLACEMENT_3D('',#43317,#33057,#33058);
#29285=AXIS2_PLACEMENT_3D('',#43319,#33060,#33061);
#29286=AXIS2_PLACEMENT_3D('',#43325,#33065,#33066);
#29287=AXIS2_PLACEMENT_3D('',#43328,#33068,#33069);
#29288=AXIS2_PLACEMENT_3D('',#43329,#33070,#33071);
#29289=AXIS2_PLACEMENT_3D('',#43333,#33074,#33075);
#29290=AXIS2_PLACEMENT_3D('',#43334,#33076,#33077);
#29291=AXIS2_PLACEMENT_3D('',#43335,#33078,#33079);
#29292=AXIS2_PLACEMENT_3D('',#43339,#33081,#33082);
#29293=AXIS2_PLACEMENT_3D('',#43341,#33084,#33085);
#29294=AXIS2_PLACEMENT_3D('',#43345,#33088,#33089);
#29295=AXIS2_PLACEMENT_3D('',#43348,#33092,#33093);
#29296=AXIS2_PLACEMENT_3D('',#43351,#33095,#33096);
#29297=AXIS2_PLACEMENT_3D('',#43352,#33097,#33098);
#29298=AXIS2_PLACEMENT_3D('',#43355,#33101,#33102);
#29299=AXIS2_PLACEMENT_3D('',#43356,#33103,#33104);
#29300=AXIS2_PLACEMENT_3D('',#43358,#33106,#33107);
#29301=AXIS2_PLACEMENT_3D('',#43359,#33108,#33109);
#29302=AXIS2_PLACEMENT_3D('',#43360,#33110,#33111);
#29303=AXIS2_PLACEMENT_3D('',#43361,#33112,#33113);
#29304=AXIS2_PLACEMENT_3D('',#43362,#33114,#33115);
#29305=AXIS2_PLACEMENT_3D('',#43363,#33116,#33117);
#32604=DIRECTION('axis',(0.,0.,1.));
#32605=DIRECTION('refdir',(1.,0.,0.));
#32606=DIRECTION('center_axis',(-0.707106781186548,0.,-0.707106781186548));
#32607=DIRECTION('ref_axis',(-0.707106781186548,0.,0.707106781186548));
#32608=DIRECTION('',(-0.707106781186548,0.,0.707106781186548));
#32609=DIRECTION('',(0.,-1.,0.));
#32610=DIRECTION('',(0.707106781186548,0.,-0.707106781186548));
#32611=DIRECTION('',(0.,1.,0.));
#32612=DIRECTION('center_axis',(0.,0.,1.));
#32613=DIRECTION('ref_axis',(1.,0.,0.));
#32614=DIRECTION('',(-1.,0.,0.));
#32615=DIRECTION('',(0.,1.,0.));
#32616=DIRECTION('',(1.,0.,0.));
#32617=DIRECTION('center_axis',(0.,0.707106781186529,-0.707106781186566));
#32618=DIRECTION('ref_axis',(-1.,0.,0.));
#32619=DIRECTION('',(-0.577350269189616,-0.577350269189646,-0.577350269189616));
#32620=DIRECTION('',(-1.,0.,0.));
#32621=DIRECTION('',(-0.577350269189616,0.577350269189646,0.577350269189616));
#32622=DIRECTION('',(0.577350269189616,0.577350269189646,0.577350269189616));
#32623=DIRECTION('',(1.,0.,0.));
#32624=DIRECTION('',(0.577350269189616,-0.577350269189646,-0.577350269189616));
#32625=DIRECTION('center_axis',(0.,1.,0.));
#32626=DIRECTION('ref_axis',(0.,0.,1.));
#32627=DIRECTION('',(0.,0.,-1.));
#32628=DIRECTION('',(-1.,0.,0.));
#32629=DIRECTION('',(0.,0.,1.));
#32630=DIRECTION('center_axis',(-0.707106781186566,0.707106781186529,0.));
#32631=DIRECTION('ref_axis',(0.,0.,1.));
#32632=DIRECTION('',(0.577350269189616,0.577350269189646,-0.577350269189616));
#32633=DIRECTION('',(0.,0.,1.));
#32634=DIRECTION('',(-0.577350269189616,-0.577350269189646,-0.577350269189616));
#32635=DIRECTION('',(-0.577350269189616,-0.577350269189646,0.577350269189616));
#32636=DIRECTION('center_axis',(-0.707106781186548,0.,-0.707106781186548));
#32637=DIRECTION('ref_axis',(-0.707106781186548,0.,0.707106781186548));
#32638=DIRECTION('',(0.,-1.,0.));
#32639=DIRECTION('',(0.577350269189616,0.577350269189646,-0.577350269189616));
#32640=DIRECTION('',(0.577350269189616,-0.577350269189646,-0.577350269189616));
#32641=DIRECTION('',(0.,1.,0.));
#32642=DIRECTION('center_axis',(-0.707106781186522,0.,0.707106781186573));
#32643=DIRECTION('ref_axis',(0.707106781186573,0.,0.707106781186522));
#32644=DIRECTION('',(0.707106781186573,0.,0.707106781186522));
#32645=DIRECTION('',(0.,-1.,0.));
#32646=DIRECTION('',(-0.707106781186573,0.,-0.707106781186522));
#32647=DIRECTION('',(0.,1.,0.));
#32648=DIRECTION('center_axis',(-1.,0.,0.));
#32649=DIRECTION('ref_axis',(0.,-1.,0.));
#32650=DIRECTION('',(0.,0.,-1.));
#32651=DIRECTION('',(0.,0.,1.));
#32652=DIRECTION('center_axis',(0.707106781186548,0.,-0.707106781186548));
#32653=DIRECTION('ref_axis',(-0.707106781186548,0.,-0.707106781186548));
#32654=DIRECTION('',(0.707106781186548,0.,0.707106781186548));
#32655=DIRECTION('',(0.,1.,0.));
#32656=DIRECTION('',(-0.707106781186548,0.,-0.707106781186548));
#32657=DIRECTION('',(0.,-1.,0.));
#32658=DIRECTION('center_axis',(0.,0.,1.));
#32659=DIRECTION('ref_axis',(1.,0.,0.));
#32660=DIRECTION('',(1.,0.,0.));
#32661=DIRECTION('',(0.,-1.,0.));
#32662=DIRECTION('',(-1.,0.,0.));
#32663=DIRECTION('center_axis',(0.,-0.707106781186529,0.707106781186566));
#32664=DIRECTION('ref_axis',(1.,0.,0.));
#32665=DIRECTION('',(-0.577350269189616,0.577350269189646,0.577350269189616));
#32666=DIRECTION('',(-1.,0.,0.));
#32667=DIRECTION('',(-0.577350269189643,-0.577350269189633,-0.577350269189602));
#32668=DIRECTION('',(0.577350269189643,-0.577350269189633,-0.577350269189602));
#32669=DIRECTION('',(1.,0.,0.));
#32670=DIRECTION('',(0.577350269189616,0.577350269189646,0.577350269189616));
#32671=DIRECTION('center_axis',(0.707106781186566,-0.707106781186529,0.));
#32672=DIRECTION('ref_axis',(0.,0.,-1.));
#32673=DIRECTION('',(0.,0.,-1.));
#32674=DIRECTION('',(-0.577350269189616,-0.577350269189646,0.577350269189616));
#32675=DIRECTION('',(-0.577350269189616,-0.577350269189646,-0.577350269189616));
#32676=DIRECTION('',(0.,0.,1.));
#32677=DIRECTION('',(0.577350269189616,0.577350269189646,-0.577350269189616));
#32678=DIRECTION('center_axis',(0.,-1.,0.));
#32679=DIRECTION('ref_axis',(0.,0.,-1.));
#32680=DIRECTION('',(0.,0.,1.));
#32681=DIRECTION('',(-1.,0.,0.));
#32682=DIRECTION('center_axis',(-0.707106781186541,-0.707106781186554,0.));
#32683=DIRECTION('ref_axis',(0.,0.,1.));
#32684=DIRECTION('',(0.577350269189643,-0.577350269189633,0.577350269189602));
#32685=DIRECTION('',(0.,0.,-1.));
#32686=DIRECTION('',(-0.577350269189643,0.577350269189633,0.577350269189602));
#32687=DIRECTION('',(-0.577350269189643,0.577350269189633,-0.577350269189602));
#32688=DIRECTION('center_axis',(0.,-0.707106781186529,-0.707106781186566));
#32689=DIRECTION('ref_axis',(-1.,0.,0.));
#32690=DIRECTION('',(0.577350269189643,0.577350269189633,-0.577350269189602));
#32691=DIRECTION('',(1.,0.,0.));
#32692=DIRECTION('',(0.577350269189616,-0.577350269189646,0.577350269189616));
#32693=DIRECTION('center_axis',(0.707106781186548,0.,-0.707106781186548));
#32694=DIRECTION('ref_axis',(-0.707106781186548,0.,-0.707106781186548));
#32695=DIRECTION('',(0.,1.,0.));
#32696=DIRECTION('',(0.707106781186548,0.,0.707106781186548));
#32697=DIRECTION('',(0.,-1.,0.));
#32698=DIRECTION('center_axis',(0.,0.,-1.));
#32699=DIRECTION('ref_axis',(0.,1.,0.));
#32700=DIRECTION('',(0.,-1.,0.));
#32701=DIRECTION('',(-1.,0.,0.));
#32702=DIRECTION('center_axis',(-0.707106781186522,0.,-0.707106781186573));
#32703=DIRECTION('ref_axis',(-0.707106781186573,0.,0.707106781186522));
#32704=DIRECTION('',(0.,1.,0.));
#32705=DIRECTION('',(0.577350269189643,0.577350269189633,-0.577350269189602));
#32706=DIRECTION('',(-0.577350269189643,0.577350269189633,0.577350269189602));
#32707=DIRECTION('center_axis',(0.707106781186548,0.,0.707106781186548));
#32708=DIRECTION('ref_axis',(0.707106781186548,0.,-0.707106781186548));
#32709=DIRECTION('',(0.,1.,0.));
#32710=DIRECTION('',(-0.577350269189614,-0.57735026918965,0.577350269189614));
#32711=DIRECTION('',(0.,-1.,0.));
#32712=DIRECTION('center_axis',(0.70710678118657,-0.707106781186526,0.));
#32713=DIRECTION('ref_axis',(0.,0.,-1.));
#32714=DIRECTION('',(0.,0.,1.));
#32715=DIRECTION('',(0.577350269189614,0.57735026918965,0.577350269189614));
#32716=DIRECTION('',(0.,0.,-1.));
#32717=DIRECTION('center_axis',(0.,0.,1.));
#32718=DIRECTION('ref_axis',(0.,-1.,0.));
#32719=DIRECTION('',(1.,0.,0.));
#32720=DIRECTION('',(0.,1.,0.));
#32721=DIRECTION('center_axis',(0.,-1.,0.));
#32722=DIRECTION('ref_axis',(0.,0.,-1.));
#32723=DIRECTION('',(1.,0.,0.));
#32724=DIRECTION('',(0.,0.,1.));
#32725=DIRECTION('center_axis',(0.707106781186522,0.,0.707106781186573));
#32726=DIRECTION('ref_axis',(0.707106781186573,0.,-0.707106781186522));
#32727=DIRECTION('',(-0.707106781186573,0.,0.707106781186522));
#32728=DIRECTION('',(0.,1.,0.));
#32729=DIRECTION('',(0.707106781186573,0.,-0.707106781186522));
#32730=DIRECTION('',(0.,-1.,0.));
#32731=DIRECTION('center_axis',(1.,0.,0.));
#32732=DIRECTION('ref_axis',(0.,1.,0.));
#32733=DIRECTION('',(0.,0.,-1.));
#32734=DIRECTION('',(0.,0.,1.));
#32735=DIRECTION('center_axis',(0.577350269189636,0.577350269189605,-0.577350269189636));
#32736=DIRECTION('ref_axis',(-0.707106781186548,0.,-0.707106781186548));
#32737=DIRECTION('',(0.,-0.707106781186566,-0.707106781186529));
#32738=DIRECTION('',(-0.707106781186529,0.707106781186566,0.));
#32739=DIRECTION('center_axis',(0.,0.707106781186529,-0.707106781186566));
#32740=DIRECTION('ref_axis',(-1.,0.,0.));
#32741=DIRECTION('',(0.577350269189643,0.577350269189633,0.577350269189602));
#32742=DIRECTION('',(1.,0.,0.));
#32743=DIRECTION('center_axis',(0.577350269189636,-0.577350269189605,-0.577350269189636));
#32744=DIRECTION('ref_axis',(-0.707106781186548,0.,-0.707106781186548));
#32745=DIRECTION('',(0.707106781186529,0.707106781186566,0.));
#32746=DIRECTION('',(0.,-0.707106781186566,0.707106781186529));
#32747=DIRECTION('',(-0.707106781186548,0.,-0.707106781186548));
#32748=DIRECTION('center_axis',(0.,-0.707106781186529,-0.707106781186566));
#32749=DIRECTION('ref_axis',(-1.,0.,0.));
#32750=DIRECTION('',(1.,0.,0.));
#32751=DIRECTION('',(-1.,0.,0.));
#32752=DIRECTION('',(-0.577350269189616,0.577350269189646,-0.577350269189616));
#32753=DIRECTION('center_axis',(0.707106781186548,0.,-0.707106781186548));
#32754=DIRECTION('ref_axis',(-0.707106781186548,0.,-0.707106781186548));
#32755=DIRECTION('',(0.577350269189616,-0.577350269189646,0.577350269189616));
#32756=DIRECTION('',(0.,-1.,0.));
#32757=DIRECTION('',(0.,1.,0.));
#32758=DIRECTION('center_axis',(0.707106781186566,-0.707106781186529,0.));
#32759=DIRECTION('ref_axis',(0.,0.,-1.));
#32760=DIRECTION('',(0.,0.,-1.));
#32761=DIRECTION('',(0.,0.,1.));
#32762=DIRECTION('',(-0.577350269189616,-0.577350269189646,-0.577350269189616));
#32763=DIRECTION('center_axis',(0.707106781186548,0.,-0.707106781186548));
#32764=DIRECTION('ref_axis',(-0.707106781186548,0.,-0.707106781186548));
#32765=DIRECTION('',(0.,-1.,0.));
#32766=DIRECTION('',(-0.577350269189616,0.577350269189646,-0.577350269189616));
#32767=DIRECTION('center_axis',(0.707106781186566,0.707106781186529,0.));
#32768=DIRECTION('ref_axis',(0.,0.,-1.));
#32769=DIRECTION('',(0.,0.,-1.));
#32770=DIRECTION('',(0.,0.,1.));
#32771=DIRECTION('center_axis',(-0.707106781186541,0.707106781186554,0.));
#32772=DIRECTION('ref_axis',(0.,0.,1.));
#32773=DIRECTION('',(0.,0.,1.));
#32774=DIRECTION('',(0.577350269189616,0.577350269189646,-0.577350269189616));
#32775=DIRECTION('',(0.,0.,-1.));
#32776=DIRECTION('center_axis',(1.,0.,0.));
#32777=DIRECTION('ref_axis',(0.,0.,-1.));
#32778=DIRECTION('',(0.,0.,-1.));
#32779=DIRECTION('',(0.,1.,0.));
#32780=DIRECTION('',(0.,0.,-1.));
#32781=DIRECTION('',(0.,-1.,0.));
#32782=DIRECTION('',(0.,0.,-1.));
#32783=DIRECTION('',(0.,1.,0.));
#32784=DIRECTION('',(0.,0.,1.));
#32785=DIRECTION('',(0.,1.,0.));
#32786=DIRECTION('',(0.,0.,-1.));
#32787=DIRECTION('',(0.,1.,0.));
#32788=DIRECTION('',(0.,0.,1.));
#32789=DIRECTION('',(0.,-1.,0.));
#32790=DIRECTION('center_axis',(0.,0.707106781186529,0.707106781186566));
#32791=DIRECTION('ref_axis',(1.,0.,0.));
#32792=DIRECTION('',(-0.577350269189616,0.577350269189646,-0.577350269189616));
#32793=DIRECTION('',(0.577350269189616,-0.577350269189646,0.577350269189616));
#32794=DIRECTION('',(1.,0.,0.));
#32795=DIRECTION('',(0.577350269189616,0.577350269189646,-0.577350269189616));
#32796=DIRECTION('center_axis',(0.707106781186548,0.,0.707106781186548));
#32797=DIRECTION('ref_axis',(0.707106781186548,0.,-0.707106781186548));
#32798=DIRECTION('',(0.,-1.,0.));
#32799=DIRECTION('',(-0.577350269189616,0.577350269189646,0.577350269189616));
#32800=DIRECTION('',(-0.577350269189616,0.577350269189646,0.577350269189616));
#32801=DIRECTION('center_axis',(0.,0.,1.));
#32802=DIRECTION('ref_axis',(0.,-1.,0.));
#32803=DIRECTION('',(0.,1.,0.));
#32804=DIRECTION('',(1.,0.,0.));
#32805=DIRECTION('center_axis',(-0.707106781186548,0.,0.707106781186548));
#32806=DIRECTION('ref_axis',(0.707106781186548,0.,0.707106781186548));
#32807=DIRECTION('',(0.,-1.,0.));
#32808=DIRECTION('',(0.577350269189614,0.57735026918965,0.577350269189614));
#32809=DIRECTION('center_axis',(0.707106781186566,0.707106781186529,0.));
#32810=DIRECTION('ref_axis',(0.,0.,-1.));
#32811=DIRECTION('',(0.,0.,1.));
#32812=DIRECTION('',(-0.577350269189616,0.577350269189646,-0.577350269189616));
#32813=DIRECTION('center_axis',(0.707106781186566,0.707106781186529,0.));
#32814=DIRECTION('ref_axis',(0.,0.,-1.));
#32815=DIRECTION('',(0.,0.,1.));
#32816=DIRECTION('',(0.577350269189616,-0.577350269189646,0.577350269189616));
#32817=DIRECTION('',(0.577350269189616,-0.577350269189646,-0.577350269189616));
#32818=DIRECTION('',(-0.577350269189616,0.577350269189646,0.577350269189616));
#32819=DIRECTION('center_axis',(0.707106781186522,0.,0.707106781186573));
#32820=DIRECTION('ref_axis',(0.707106781186573,0.,-0.707106781186522));
#32821=DIRECTION('',(-0.577350269189616,-0.577350269189646,0.577350269189616));
#32822=DIRECTION('',(0.,-1.,0.));
#32823=DIRECTION('center_axis',(0.577350269189636,-0.577350269189605,0.577350269189636));
#32824=DIRECTION('ref_axis',(0.707106781186548,0.,-0.707106781186548));
#32825=DIRECTION('',(0.707106781186548,0.,-0.707106781186548));
#32826=DIRECTION('',(0.,0.707106781186566,0.707106781186529));
#32827=DIRECTION('',(-0.707106781186529,-0.707106781186566,0.));
#32828=DIRECTION('center_axis',(0.,-0.707106781186529,0.707106781186566));
#32829=DIRECTION('ref_axis',(1.,0.,0.));
#32830=DIRECTION('',(0.577350269189616,-0.577350269189646,-0.577350269189616));
#32831=DIRECTION('',(1.,0.,0.));
#32832=DIRECTION('',(-1.,0.,0.));
#32833=DIRECTION('',(-0.577350269189616,-0.577350269189646,-0.577350269189616));
#32834=DIRECTION('center_axis',(0.707106781186566,-0.707106781186529,0.));
#32835=DIRECTION('ref_axis',(0.,0.,-1.));
#32836=DIRECTION('',(0.,0.,-1.));
#32837=DIRECTION('center_axis',(0.707106781186548,0.,0.707106781186548));
#32838=DIRECTION('ref_axis',(0.707106781186548,0.,-0.707106781186548));
#32839=DIRECTION('',(-0.577350269189616,-0.577350269189646,0.577350269189616));
#32840=DIRECTION('',(0.,-1.,0.));
#32841=DIRECTION('',(-0.577350269189616,0.577350269189646,0.577350269189616));
#32842=DIRECTION('center_axis',(0.,0.,1.));
#32843=DIRECTION('ref_axis',(1.,0.,0.));
#32844=DIRECTION('',(-1.,0.,0.));
#32845=DIRECTION('',(1.,0.,0.));
#32846=DIRECTION('center_axis',(0.,-1.,0.));
#32847=DIRECTION('ref_axis',(0.,0.,-1.));
#32848=DIRECTION('',(0.,0.,1.));
#32849=DIRECTION('',(1.,0.,0.));
#32850=DIRECTION('',(0.,0.,1.));
#32851=DIRECTION('center_axis',(-0.707106781186566,-0.707106781186529,0.));
#32852=DIRECTION('ref_axis',(0.,0.,1.));
#32853=DIRECTION('',(0.577350269189616,-0.577350269189646,0.577350269189616));
#32854=DIRECTION('',(0.,0.,-1.));
#32855=DIRECTION('',(0.577350269189616,-0.577350269189646,0.577350269189616));
#32856=DIRECTION('center_axis',(-0.707106781186548,0.,0.707106781186548));
#32857=DIRECTION('ref_axis',(0.707106781186548,0.,0.707106781186548));
#32858=DIRECTION('',(0.,1.,0.));
#32859=DIRECTION('',(0.577350269189616,-0.577350269189646,0.577350269189616));
#32860=DIRECTION('',(-0.577350269189616,-0.577350269189646,-0.577350269189616));
#32861=DIRECTION('',(0.,-1.,0.));
#32862=DIRECTION('center_axis',(0.,0.,1.));
#32863=DIRECTION('ref_axis',(0.,-1.,0.));
#32864=DIRECTION('',(1.,0.,0.));
#32865=DIRECTION('',(1.,0.,0.));
#32866=DIRECTION('center_axis',(0.,0.,1.));
#32867=DIRECTION('ref_axis',(0.,1.,0.));
#32868=DIRECTION('',(-1.,0.,0.));
#32869=DIRECTION('center_axis',(0.,0.,1.));
#32870=DIRECTION('ref_axis',(0.,-1.,0.));
#32871=DIRECTION('center_axis',(0.,0.707106781186529,0.707106781186566));
#32872=DIRECTION('ref_axis',(1.,0.,0.));
#32873=DIRECTION('',(-0.577350269189616,0.577350269189646,-0.577350269189616));
#32874=DIRECTION('',(-1.,0.,0.));
#32875=DIRECTION('',(-0.577350269189616,-0.577350269189646,0.577350269189616));
#32876=DIRECTION('center_axis',(-0.707106781186566,0.707106781186529,0.));
#32877=DIRECTION('ref_axis',(0.,0.,1.));
#32878=DIRECTION('',(0.,0.,-1.));
#32879=DIRECTION('',(0.577350269189616,0.577350269189646,0.577350269189616));
#32880=DIRECTION('',(0.577350269189616,0.577350269189646,-0.577350269189616));
#32881=DIRECTION('',(0.,0.,1.));
#32882=DIRECTION('center_axis',(0.,0.707106781186529,-0.707106781186566));
#32883=DIRECTION('ref_axis',(-1.,0.,0.));
#32884=DIRECTION('',(-0.577350269189616,-0.577350269189646,-0.577350269189616));
#32885=DIRECTION('',(-1.,0.,0.));
#32886=DIRECTION('',(-0.577350269189616,0.577350269189646,0.577350269189616));
#32887=DIRECTION('',(1.,0.,0.));
#32888=DIRECTION('',(0.577350269189616,-0.577350269189646,-0.577350269189616));
#32889=DIRECTION('center_axis',(-0.707106781186548,0.,-0.707106781186548));
#32890=DIRECTION('ref_axis',(-0.707106781186548,0.,0.707106781186548));
#32891=DIRECTION('',(0.,-1.,0.));
#32892=DIRECTION('',(0.577350269189614,0.57735026918965,-0.577350269189614));
#32893=DIRECTION('',(0.,1.,0.));
#32894=DIRECTION('center_axis',(0.,0.,-1.));
#32895=DIRECTION('ref_axis',(0.,1.,0.));
#32896=DIRECTION('',(0.,1.,0.));
#32897=DIRECTION('',(1.,0.,0.));
#32898=DIRECTION('',(-1.,0.,0.));
#32899=DIRECTION('center_axis',(0.,0.,-1.));
#32900=DIRECTION('ref_axis',(0.,-1.,0.));
#32901=DIRECTION('',(1.,0.,0.));
#32902=DIRECTION('center_axis',(0.,0.,-1.));
#32903=DIRECTION('ref_axis',(0.,1.,0.));
#32904=DIRECTION('center_axis',(0.707106781186548,0.,-0.707106781186548));
#32905=DIRECTION('ref_axis',(-0.707106781186548,0.,-0.707106781186548));
#32906=DIRECTION('',(0.577350269189616,-0.577350269189646,0.577350269189616));
#32907=DIRECTION('center_axis',(0.707106781186566,0.707106781186529,0.));
#32908=DIRECTION('ref_axis',(0.,0.,-1.));
#32909=DIRECTION('',(0.,0.,1.));
#32910=DIRECTION('center_axis',(-0.707106781186548,0.,-0.707106781186548));
#32911=DIRECTION('ref_axis',(-0.707106781186548,0.,0.707106781186548));
#32912=DIRECTION('',(0.,1.,0.));
#32913=DIRECTION('',(0.577350269189616,-0.577350269189646,-0.577350269189616));
#32914=DIRECTION('center_axis',(-0.707106781186566,-0.707106781186529,0.));
#32915=DIRECTION('ref_axis',(0.,0.,1.));
#32916=DIRECTION('',(0.,0.,-1.));
#32917=DIRECTION('center_axis',(1.,0.,0.));
#32918=DIRECTION('ref_axis',(0.,0.,-1.));
#32919=DIRECTION('',(0.,-1.,0.));
#32920=DIRECTION('',(0.,0.,-1.));
#32921=DIRECTION('',(0.,1.,0.));
#32922=DIRECTION('',(0.,0.,-1.));
#32923=DIRECTION('',(0.,-1.,0.));
#32924=DIRECTION('',(0.,0.,1.));
#32925=DIRECTION('',(0.,-1.,0.));
#32926=DIRECTION('',(0.,0.,1.));
#32927=DIRECTION('center_axis',(-0.70710678118657,0.707106781186526,0.));
#32928=DIRECTION('ref_axis',(0.,0.,1.));
#32929=DIRECTION('',(0.,0.,-1.));
#32930=DIRECTION('center_axis',(0.,1.,0.));
#32931=DIRECTION('ref_axis',(0.,0.,1.));
#32932=DIRECTION('center_axis',(-0.577350269189609,0.577350269189619,0.57735026918965));
#32933=DIRECTION('ref_axis',(0.707106781186573,0.,0.707106781186523));
#32934=DIRECTION('',(0.,-0.707106781186566,0.707106781186529));
#32935=DIRECTION('',(0.707106781186554,0.707106781186541,0.));
#32936=DIRECTION('',(-0.707106781186573,0.,-0.707106781186522));
#32937=DIRECTION('center_axis',(-0.707106781186541,0.707106781186554,0.));
#32938=DIRECTION('ref_axis',(0.,0.,1.));
#32939=DIRECTION('',(0.,0.,-1.));
#32940=DIRECTION('',(-0.577350269189643,-0.577350269189633,-0.577350269189602));
#32941=DIRECTION('center_axis',(-0.707106781186522,0.,0.707106781186573));
#32942=DIRECTION('ref_axis',(0.707106781186573,0.,0.707106781186522));
#32943=DIRECTION('',(0.577350269189643,0.577350269189633,0.577350269189602));
#32944=DIRECTION('',(0.,1.,0.));
#32945=DIRECTION('',(0.577350269189643,-0.577350269189633,0.577350269189602));
#32946=DIRECTION('center_axis',(0.,0.707106781186529,0.707106781186566));
#32947=DIRECTION('ref_axis',(1.,0.,0.));
#32948=DIRECTION('',(-1.,0.,0.));
#32949=DIRECTION('',(1.,0.,0.));
#32950=DIRECTION('',(0.577350269189616,0.577350269189646,-0.577350269189616));
#32951=DIRECTION('center_axis',(-0.707106781186522,0.,0.707106781186573));
#32952=DIRECTION('ref_axis',(0.707106781186573,0.,0.707106781186522));
#32953=DIRECTION('',(0.,1.,0.));
#32954=DIRECTION('center_axis',(0.707106781186548,0.,0.707106781186548));
#32955=DIRECTION('ref_axis',(0.707106781186548,0.,-0.707106781186548));
#32956=DIRECTION('',(0.,-1.,0.));
#32957=DIRECTION('',(0.577350269189616,-0.577350269189646,-0.577350269189616));
#32958=DIRECTION('',(0.577350269189616,0.577350269189646,-0.577350269189616));
#32959=DIRECTION('center_axis',(0.,0.,1.));
#32960=DIRECTION('ref_axis',(1.,0.,0.));
#32961=DIRECTION('',(-1.,0.,0.));
#32962=DIRECTION('center_axis',(0.,1.,0.));
#32963=DIRECTION('ref_axis',(0.,0.,1.));
#32964=DIRECTION('center_axis',(0.707106781186566,-0.707106781186529,0.));
#32965=DIRECTION('ref_axis',(0.,0.,-1.));
#32966=DIRECTION('',(0.577350269189616,0.577350269189646,0.577350269189616));
#32967=DIRECTION('',(0.,0.,-1.));
#32968=DIRECTION('',(-0.577350269189616,-0.577350269189646,0.577350269189616));
#32969=DIRECTION('',(-0.577350269189616,-0.577350269189646,-0.577350269189616));
#32970=DIRECTION('center_axis',(-0.707106781186544,-0.707106781186551,0.));
#32971=DIRECTION('ref_axis',(0.,0.,1.));
#32972=DIRECTION('',(0.577350269189641,-0.577350269189636,-0.5773502691896));
#32973=DIRECTION('',(0.577350269189641,-0.577350269189636,0.5773502691896));
#32974=DIRECTION('center_axis',(-0.707106781186522,0.,0.707106781186573));
#32975=DIRECTION('ref_axis',(0.707106781186573,0.,0.707106781186522));
#32976=DIRECTION('center_axis',(0.707106781186548,0.,-0.707106781186548));
#32977=DIRECTION('ref_axis',(-0.707106781186548,0.,-0.707106781186548));
#32978=DIRECTION('',(-0.577350269189616,0.577350269189646,-0.577350269189616));
#32979=DIRECTION('',(0.,1.,0.));
#32980=DIRECTION('center_axis',(0.,0.,-1.));
#32981=DIRECTION('ref_axis',(0.,1.,0.));
#32982=DIRECTION('',(1.,0.,0.));
#32983=DIRECTION('',(0.,-1.,0.));
#32984=DIRECTION('',(-1.,0.,0.));
#32985=DIRECTION('center_axis',(0.,0.,-1.));
#32986=DIRECTION('ref_axis',(0.,-1.,0.));
#32987=DIRECTION('',(1.,0.,0.));
#32988=DIRECTION('center_axis',(0.,0.,-1.));
#32989=DIRECTION('ref_axis',(0.,1.,0.));
#32990=DIRECTION('center_axis',(0.,-0.707106781186529,-0.707106781186566));
#32991=DIRECTION('ref_axis',(-1.,0.,0.));
#32992=DIRECTION('',(-1.,0.,0.));
#32993=DIRECTION('',(-0.577350269189643,0.577350269189633,-0.577350269189602));
#32994=DIRECTION('',(-0.577350269189643,-0.577350269189633,0.577350269189602));
#32995=DIRECTION('center_axis',(-0.707106781186522,0.,-0.707106781186573));
#32996=DIRECTION('ref_axis',(-0.707106781186573,0.,0.707106781186522));
#32997=DIRECTION('',(-0.577350269189643,0.577350269189633,0.577350269189602));
#32998=DIRECTION('center_axis',(-0.707106781186541,-0.707106781186554,0.));
#32999=DIRECTION('ref_axis',(0.,0.,1.));
#33000=DIRECTION('',(0.,0.,1.));
#33001=DIRECTION('',(0.577350269189643,-0.577350269189633,-0.577350269189602));
#33002=DIRECTION('center_axis',(0.,-0.707106781186529,0.707106781186566));
#33003=DIRECTION('ref_axis',(1.,0.,0.));
#33004=DIRECTION('',(1.,0.,0.));
#33005=DIRECTION('',(-1.,0.,0.));
#33006=DIRECTION('center_axis',(0.,0.,1.));
#33007=DIRECTION('ref_axis',(0.,-1.,0.));
#33008=DIRECTION('',(1.,0.,0.));
#33009=DIRECTION('center_axis',(0.,0.,1.));
#33010=DIRECTION('ref_axis',(0.,1.,0.));
#33011=DIRECTION('',(-1.,0.,0.));
#33012=DIRECTION('center_axis',(0.,0.,1.));
#33013=DIRECTION('ref_axis',(0.,-1.,0.));
#33014=DIRECTION('center_axis',(0.,0.707106781186529,-0.707106781186566));
#33015=DIRECTION('ref_axis',(-1.,0.,0.));
#33016=DIRECTION('',(0.,-0.707106781186566,-0.707106781186529));
#33017=DIRECTION('',(0.,0.70710678118657,0.707106781186526));
#33018=DIRECTION('',(1.,0.,0.));
#33019=DIRECTION('center_axis',(0.,0.,-1.));
#33020=DIRECTION('ref_axis',(0.,-1.,0.));
#33021=DIRECTION('',(0.,0.70710678118657,-0.707106781186526));
#33022=DIRECTION('center_axis',(0.,0.,1.));
#33023=DIRECTION('ref_axis',(0.,-1.,0.));
#33024=DIRECTION('center_axis',(0.,-0.707106781186529,-0.707106781186566));
#33025=DIRECTION('ref_axis',(-1.,0.,0.));
#33026=DIRECTION('',(0.,0.707106781186566,-0.707106781186529));
#33027=DIRECTION('',(-1.,0.,0.));
#33028=DIRECTION('center_axis',(0.,0.,-1.));
#33029=DIRECTION('ref_axis',(0.,1.,0.));
#33030=DIRECTION('center_axis',(0.,0.,1.));
#33031=DIRECTION('ref_axis',(0.,1.,0.));
#33032=DIRECTION('center_axis',(0.,0.,-1.));
#33033=DIRECTION('ref_axis',(0.,-1.,0.));
#33034=DIRECTION('',(0.,0.,-1.));
#33035=DIRECTION('center_axis',(0.,0.,-1.));
#33036=DIRECTION('ref_axis',(0.,-1.,0.));
#33037=DIRECTION('',(0.,0.,-1.));
#33038=DIRECTION('center_axis',(0.,-1.,0.));
#33039=DIRECTION('ref_axis',(-1.,0.,0.));
#33040=DIRECTION('',(0.,0.,-1.));
#33041=DIRECTION('',(-1.,0.,0.));
#33042=DIRECTION('center_axis',(0.,0.707106781186532,0.707106781186563));
#33043=DIRECTION('ref_axis',(1.,0.,0.));
#33044=DIRECTION('',(0.,-0.707106781186566,0.707106781186529));
#33045=DIRECTION('',(0.,0.707106781186563,-0.707106781186532));
#33046=DIRECTION('center_axis',(0.,0.,1.));
#33047=DIRECTION('ref_axis',(0.,1.,0.));
#33048=DIRECTION('',(0.,0.707106781186566,0.707106781186529));
#33049=DIRECTION('center_axis',(0.,0.,-1.));
#33050=DIRECTION('ref_axis',(0.,1.,0.));
#33051=DIRECTION('center_axis',(0.,-0.707106781186529,0.707106781186566));
#33052=DIRECTION('ref_axis',(1.,0.,0.));
#33053=DIRECTION('',(0.,0.707106781186566,0.707106781186529));
#33054=DIRECTION('',(1.,0.,0.));
#33055=DIRECTION('center_axis',(0.,0.,1.));
#33056=DIRECTION('ref_axis',(0.,-1.,0.));
#33057=DIRECTION('center_axis',(0.,0.,-1.));
#33058=DIRECTION('ref_axis',(0.,1.,0.));
#33059=DIRECTION('',(0.,0.,-1.));
#33060=DIRECTION('center_axis',(0.,0.707106781186529,-0.707106781186566));
#33061=DIRECTION('ref_axis',(-1.,0.,0.));
#33062=DIRECTION('',(0.,-0.707106781186566,-0.707106781186529));
#33063=DIRECTION('',(0.,0.707106781186563,0.707106781186532));
#33064=DIRECTION('',(1.,0.,0.));
#33065=DIRECTION('center_axis',(0.,0.,-1.));
#33066=DIRECTION('ref_axis',(0.,-1.,0.));
#33067=DIRECTION('',(0.,0.707106781186563,-0.707106781186532));
#33068=DIRECTION('center_axis',(0.,0.,1.));
#33069=DIRECTION('ref_axis',(0.,-1.,0.));
#33070=DIRECTION('center_axis',(0.,-0.707106781186532,-0.707106781186563));
#33071=DIRECTION('ref_axis',(-1.,0.,0.));
#33072=DIRECTION('',(0.,0.707106781186563,-0.707106781186532));
#33073=DIRECTION('',(-1.,0.,0.));
#33074=DIRECTION('center_axis',(0.,0.,-1.));
#33075=DIRECTION('ref_axis',(0.,1.,0.));
#33076=DIRECTION('center_axis',(0.,0.,1.));
#33077=DIRECTION('ref_axis',(0.,1.,0.));
#33078=DIRECTION('center_axis',(0.,0.,-1.));
#33079=DIRECTION('ref_axis',(0.,-1.,0.));
#33080=DIRECTION('',(0.,0.,-1.));
#33081=DIRECTION('center_axis',(0.,0.,-1.));
#33082=DIRECTION('ref_axis',(0.,-1.,0.));
#33083=DIRECTION('',(0.,0.,-1.));
#33084=DIRECTION('center_axis',(0.,-1.,0.));
#33085=DIRECTION('ref_axis',(-1.,0.,0.));
#33086=DIRECTION('',(0.,0.,-1.));
#33087=DIRECTION('',(-1.,0.,0.));
#33088=DIRECTION('center_axis',(0.,0.707106781186529,0.707106781186566));
#33089=DIRECTION('ref_axis',(1.,0.,0.));
#33090=DIRECTION('',(0.,-0.707106781186563,0.707106781186532));
#33091=DIRECTION('',(0.,0.707106781186566,-0.707106781186529));
#33092=DIRECTION('center_axis',(0.,0.,1.));
#33093=DIRECTION('ref_axis',(0.,1.,0.));
#33094=DIRECTION('',(0.,0.707106781186566,0.707106781186529));
#33095=DIRECTION('center_axis',(0.,0.,-1.));
#33096=DIRECTION('ref_axis',(0.,1.,0.));
#33097=DIRECTION('center_axis',(0.,-0.707106781186532,0.707106781186563));
#33098=DIRECTION('ref_axis',(1.,0.,0.));
#33099=DIRECTION('',(0.,0.707106781186563,0.707106781186532));
#33100=DIRECTION('',(1.,0.,0.));
#33101=DIRECTION('center_axis',(0.,0.,1.));
#33102=DIRECTION('ref_axis',(0.,-1.,0.));
#33103=DIRECTION('center_axis',(0.,0.,-1.));
#33104=DIRECTION('ref_axis',(0.,1.,0.));
#33105=DIRECTION('',(0.,0.,-1.));
#33106=DIRECTION('center_axis',(0.,1.,0.));
#33107=DIRECTION('ref_axis',(1.,0.,0.));
#33108=DIRECTION('center_axis',(0.,1.,0.));
#33109=DIRECTION('ref_axis',(1.,0.,0.));
#33110=DIRECTION('center_axis',(0.,-1.,0.));
#33111=DIRECTION('ref_axis',(0.,0.,-1.));
#33112=DIRECTION('center_axis',(0.707106781186566,0.707106781186529,0.));
#33113=DIRECTION('ref_axis',(0.,0.,-1.));
#33114=DIRECTION('center_axis',(0.,1.,0.));
#33115=DIRECTION('ref_axis',(0.,0.,1.));
#33116=DIRECTION('center_axis',(0.,0.,-1.));
#33117=DIRECTION('ref_axis',(0.,1.,0.));
#42803=CARTESIAN_POINT('',(0.,0.,0.));
#42804=CARTESIAN_POINT('Origin',(34.55,2.05,77.05));
#42805=CARTESIAN_POINT('',(34.5,4.1,77.1));
#42806=CARTESIAN_POINT('',(34.6,4.1,77.));
#42807=CARTESIAN_POINT('',(14.175,4.1,97.425));
#42808=CARTESIAN_POINT('',(34.6,-4.1,77.));
#42809=CARTESIAN_POINT('',(34.6,2.05,77.));
#42810=CARTESIAN_POINT('',(34.5,-4.1,77.1));
#42811=CARTESIAN_POINT('',(16.675,-4.1,94.925));
#42812=CARTESIAN_POINT('',(34.5,2.05,77.1));
#42813=CARTESIAN_POINT('Origin',(36.25,0.,77.));
#42814=CARTESIAN_POINT('',(37.9,4.1,77.));
#42815=CARTESIAN_POINT('',(-0.875,4.1,77.));
#42816=CARTESIAN_POINT('',(37.9,-4.1,77.));
#42817=CARTESIAN_POINT('',(37.9,3.3,77.));
#42818=CARTESIAN_POINT('',(-0.875,-4.1,77.));
#42819=CARTESIAN_POINT('Origin',(-38.,9.05,76.05));
#42820=CARTESIAN_POINT('',(37.95,9.05000000000001,76.05));
#42821=CARTESIAN_POINT('',(37.9,9.,76.));
#42822=CARTESIAN_POINT('',(24.6750000000004,-4.22500000000027,62.7750000000004));
#42823=CARTESIAN_POINT('',(-37.9,9.,76.));
#42824=CARTESIAN_POINT('',(-38.,9.,76.));
#42825=CARTESIAN_POINT('',(-37.95,9.05000000000001,76.05));
#42826=CARTESIAN_POINT('',(-36.2416666666666,7.34166666666655,74.3416666666666));
#42827=CARTESIAN_POINT('',(-37.9,9.1,76.1));
#42828=CARTESIAN_POINT('',(-37.55,9.45000000000001,76.45));
#42829=CARTESIAN_POINT('',(37.9,9.1,76.1));
#42830=CARTESIAN_POINT('',(-38.,9.1,76.1));
#42831=CARTESIAN_POINT('',(24.8833333333338,22.1166666666669,89.1166666666662));
#42832=CARTESIAN_POINT('Origin',(-38.,9.1,76.));
#42833=CARTESIAN_POINT('',(-37.9,9.1,76.5));
#42834=CARTESIAN_POINT('',(-37.9,9.1,78.5));
#42835=CARTESIAN_POINT('',(37.9,9.1,76.5));
#42836=CARTESIAN_POINT('',(-38.,9.1,76.5));
#42837=CARTESIAN_POINT('',(37.9,9.1,78.5));
#42838=CARTESIAN_POINT('Origin',(-37.95,9.05,78.5));
#42839=CARTESIAN_POINT('',(-38.,9.,76.1));
#42840=CARTESIAN_POINT('',(-40.075,6.92499999999987,78.175));
#42841=CARTESIAN_POINT('',(-38.,9.,76.5));
#42842=CARTESIAN_POINT('',(-38.,9.,78.5));
#42843=CARTESIAN_POINT('',(-37.95,9.04999999999999,76.55));
#42844=CARTESIAN_POINT('',(-38.925,8.07499999999991,75.575));
#42845=CARTESIAN_POINT('',(-38.2833333333333,8.71666666666666,76.8833333333333));
#42846=CARTESIAN_POINT('Origin',(-37.95,-1.25,76.05));
#42847=CARTESIAN_POINT('',(-37.9,4.2,76.));
#42848=CARTESIAN_POINT('',(-37.9,-1.25,76.));
#42849=CARTESIAN_POINT('',(-37.95,4.15,76.05));
#42850=CARTESIAN_POINT('',(-38.8583333333333,3.2416666666666,76.9583333333333));
#42851=CARTESIAN_POINT('',(-38.,4.2,76.1));
#42852=CARTESIAN_POINT('',(-38.,4.2,76.1));
#42853=CARTESIAN_POINT('',(-38.,-1.25,76.1));
#42854=CARTESIAN_POINT('Origin',(34.55,2.05,84.95));
#42855=CARTESIAN_POINT('',(34.6,4.1,85.));
#42856=CARTESIAN_POINT('',(34.5,4.1,84.9));
#42857=CARTESIAN_POINT('',(16.6749999999987,4.1,67.075));
#42858=CARTESIAN_POINT('',(34.5,-4.1,84.9));
#42859=CARTESIAN_POINT('',(34.5,2.05,84.9));
#42860=CARTESIAN_POINT('',(34.6,-4.1,85.));
#42861=CARTESIAN_POINT('',(14.1749999999987,-4.1,64.5750000000002));
#42862=CARTESIAN_POINT('',(34.6,2.05,85.));
#42863=CARTESIAN_POINT('Origin',(34.5,4.1,77.));
#42864=CARTESIAN_POINT('',(34.5,-4.1,76.5));
#42865=CARTESIAN_POINT('',(34.5,4.1,81.5));
#42866=CARTESIAN_POINT('Origin',(-34.55,-2.05,77.05));
#42867=CARTESIAN_POINT('',(-34.5,-4.1,77.1));
#42868=CARTESIAN_POINT('',(-34.6,-4.1,77.));
#42869=CARTESIAN_POINT('',(-35.675,-4.1,75.925));
#42870=CARTESIAN_POINT('',(-34.6,4.1,77.));
#42871=CARTESIAN_POINT('',(-34.6,-2.05,77.));
#42872=CARTESIAN_POINT('',(-34.5,4.1,77.1));
#42873=CARTESIAN_POINT('',(-33.175,4.1,78.425));
#42874=CARTESIAN_POINT('',(-34.5,-2.05,77.1));
#42875=CARTESIAN_POINT('Origin',(-36.25,0.,77.));
#42876=CARTESIAN_POINT('',(-37.9,-4.1,77.));
#42877=CARTESIAN_POINT('',(-37.125,-4.1,77.));
#42878=CARTESIAN_POINT('',(-37.9,4.1,77.));
#42879=CARTESIAN_POINT('',(-37.9,-3.3,77.));
#42880=CARTESIAN_POINT('',(-37.125,4.1,77.));
#42881=CARTESIAN_POINT('Origin',(-38.,-9.05,76.55));
#42882=CARTESIAN_POINT('',(37.95,-9.05,76.55));
#42883=CARTESIAN_POINT('',(37.9,-9.,76.6));
#42884=CARTESIAN_POINT('',(23.6250000000004,5.27500000000034,90.8749999999996));
#42885=CARTESIAN_POINT('',(-37.9,-9.,76.6));
#42886=CARTESIAN_POINT('',(-38.,-9.,76.6));
#42887=CARTESIAN_POINT('',(-37.95,-9.05,76.55));
#42888=CARTESIAN_POINT('',(-37.3916666666667,-8.49166666666665,77.1083333333333));
#42889=CARTESIAN_POINT('',(-37.9,-9.1,76.5));
#42890=CARTESIAN_POINT('',(-38.3333333333333,-8.66666666666668,76.9333333333333));
#42891=CARTESIAN_POINT('',(37.9,-9.1,76.5));
#42892=CARTESIAN_POINT('',(-38.,-9.1,76.5));
#42893=CARTESIAN_POINT('',(25.6666666666671,-21.3333333333336,64.2666666666671));
#42894=CARTESIAN_POINT('Origin',(37.95,-9.05,78.8));
#42895=CARTESIAN_POINT('',(37.9,-9.1,76.1));
#42896=CARTESIAN_POINT('',(37.9,-9.1,78.8));
#42897=CARTESIAN_POINT('',(37.95,-9.05,76.05));
#42898=CARTESIAN_POINT('',(24.8333333333338,-22.1666666666669,89.1666666666662));
#42899=CARTESIAN_POINT('',(38.,-9.,76.1));
#42900=CARTESIAN_POINT('',(39.7083333333333,-7.29166666666657,77.8083333333333));
#42901=CARTESIAN_POINT('',(38.,-9.,76.5));
#42902=CARTESIAN_POINT('',(38.,-9.,78.8));
#42903=CARTESIAN_POINT('',(39.2416666666667,-7.75833333333322,75.2583333333333));
#42904=CARTESIAN_POINT('Origin',(-38.,-9.1,76.6));
#42905=CARTESIAN_POINT('',(-37.9,-9.1,76.1));
#42906=CARTESIAN_POINT('',(-37.9,-9.1,78.8));
#42907=CARTESIAN_POINT('',(-38.,-9.1,76.1));
#42908=CARTESIAN_POINT('Origin',(-37.95,-9.05,78.8));
#42909=CARTESIAN_POINT('',(-38.,-9.,76.5));
#42910=CARTESIAN_POINT('',(-38.1416666666667,-8.85833333333331,76.3583333333333));
#42911=CARTESIAN_POINT('',(-38.,-9.,76.1));
#42912=CARTESIAN_POINT('',(-38.,-9.,78.8));
#42913=CARTESIAN_POINT('',(-37.95,-9.05000000000001,76.05));
#42914=CARTESIAN_POINT('',(-38.6083333333333,-8.39166666666668,76.7083333333333));
#42915=CARTESIAN_POINT('',(-37.5,-9.49999999999999,76.5));
#42916=CARTESIAN_POINT('Origin',(-38.,-9.05,76.05));
#42917=CARTESIAN_POINT('',(-37.9,-9.,76.));
#42918=CARTESIAN_POINT('',(-37.7583333333333,-8.85833333333333,75.8583333333333));
#42919=CARTESIAN_POINT('',(37.9,-9.,76.));
#42920=CARTESIAN_POINT('',(-38.,-9.,76.));
#42921=CARTESIAN_POINT('',(23.9916666666671,4.90833333333365,62.0916666666671));
#42922=CARTESIAN_POINT('Origin',(37.95,-1.25,76.05));
#42923=CARTESIAN_POINT('',(37.9,-4.2,76.));
#42924=CARTESIAN_POINT('',(37.9,-1.25,76.));
#42925=CARTESIAN_POINT('',(38.,-4.2,76.1));
#42926=CARTESIAN_POINT('',(37.9,-4.2,76.));
#42927=CARTESIAN_POINT('',(38.,-1.25,76.1));
#42928=CARTESIAN_POINT('Origin',(-38.,-9.1,76.));
#42929=CARTESIAN_POINT('',(-37.9,-4.2,76.));
#42930=CARTESIAN_POINT('',(-37.9,-7.85,76.));
#42931=CARTESIAN_POINT('',(-38.,-4.2,76.));
#42932=CARTESIAN_POINT('Origin',(-37.95,-7.85,76.05));
#42933=CARTESIAN_POINT('',(-38.,-4.2,76.1));
#42934=CARTESIAN_POINT('',(-38.,-7.85,76.1));
#42935=CARTESIAN_POINT('',(-37.95,-4.15,76.05));
#42936=CARTESIAN_POINT('',(-38.,-4.2,76.1));
#42937=CARTESIAN_POINT('',(-37.3416666666666,-4.75833333333335,75.4416666666667));
#42938=CARTESIAN_POINT('Origin',(37.95,0.95,76.55));
#42939=CARTESIAN_POINT('',(38.,-4.6,76.5));
#42940=CARTESIAN_POINT('',(38.,0.95,76.5));
#42941=CARTESIAN_POINT('',(37.9,-4.7,76.6));
#42942=CARTESIAN_POINT('',(38.,-4.6,76.5));
#42943=CARTESIAN_POINT('',(37.9,0.95,76.6));
#42944=CARTESIAN_POINT('Origin',(37.95,-4.65,83.2));
#42945=CARTESIAN_POINT('',(38.,-4.6,85.5));
#42946=CARTESIAN_POINT('',(38.,-4.6,83.2));
#42947=CARTESIAN_POINT('',(37.9,-4.7,85.4));
#42948=CARTESIAN_POINT('',(38.1416666666667,-4.45833333333329,85.6416666666667));
#42949=CARTESIAN_POINT('',(37.9,-4.7,83.2));
#42950=CARTESIAN_POINT('Origin',(-38.,-4.7,76.6));
#42951=CARTESIAN_POINT('',(-37.9,-4.7,76.6));
#42952=CARTESIAN_POINT('',(-38.,-4.7,76.6));
#42953=CARTESIAN_POINT('',(-37.9,-5.65,76.6));
#42954=CARTESIAN_POINT('Origin',(-38.,-4.7,85.4));
#42955=CARTESIAN_POINT('',(-37.9,-4.7,85.4));
#42956=CARTESIAN_POINT('',(-38.,-4.7,85.4));
#42957=CARTESIAN_POINT('',(-37.9,-4.7,83.2));
#42958=CARTESIAN_POINT('Origin',(-34.55,-2.05,84.95));
#42959=CARTESIAN_POINT('',(-34.6,-4.1,85.));
#42960=CARTESIAN_POINT('',(-34.5,-4.1,84.9));
#42961=CARTESIAN_POINT('',(-33.1750000000001,-4.1,83.5750000000002));
#42962=CARTESIAN_POINT('',(-34.5,4.1,84.9));
#42963=CARTESIAN_POINT('',(-34.5,-2.05,84.9));
#42964=CARTESIAN_POINT('',(-34.6,4.1,85.));
#42965=CARTESIAN_POINT('',(-35.6750000000001,4.1,86.075));
#42966=CARTESIAN_POINT('',(-34.6,-2.05,85.));
#42967=CARTESIAN_POINT('Origin',(-34.5,-4.1,77.));
#42968=CARTESIAN_POINT('',(-34.5,4.1,81.5));
#42969=CARTESIAN_POINT('',(-34.5,-4.1,76.5));
#42970=CARTESIAN_POINT('Origin',(37.9,-4.1,76.1));
#42971=CARTESIAN_POINT('',(37.9,-4.1,76.1));
#42972=CARTESIAN_POINT('',(37.9,-4.1,76.1));
#42973=CARTESIAN_POINT('',(38.,-4.2,76.1));
#42974=CARTESIAN_POINT('Origin',(-38.,-4.15,76.05));
#42975=CARTESIAN_POINT('',(-37.9,-4.1,76.1));
#42976=CARTESIAN_POINT('',(-37.55,-3.75000000000001,76.45));
#42977=CARTESIAN_POINT('',(-38.,-4.1,76.1));
#42978=CARTESIAN_POINT('Origin',(37.9,4.2,76.));
#42979=CARTESIAN_POINT('',(37.9,4.1,76.1));
#42980=CARTESIAN_POINT('',(38.,4.2,76.1));
#42981=CARTESIAN_POINT('',(37.9,4.1,76.1));
#42982=CARTESIAN_POINT('',(37.9,4.2,76.));
#42983=CARTESIAN_POINT('',(37.9,4.2,76.));
#42984=CARTESIAN_POINT('',(38.,4.2,76.1));
#42985=CARTESIAN_POINT('Origin',(-38.,4.15,76.05));
#42986=CARTESIAN_POINT('',(-38.,4.2,76.));
#42987=CARTESIAN_POINT('',(-37.9,4.1,76.1));
#42988=CARTESIAN_POINT('',(-38.,4.1,76.1));
#42989=CARTESIAN_POINT('',(-36.7166666666667,2.91666666666664,77.2833333333333));
#42990=CARTESIAN_POINT('Origin',(37.95,5.35,76.05));
#42991=CARTESIAN_POINT('',(38.,9.,76.1));
#42992=CARTESIAN_POINT('',(38.975,8.02499999999995,77.075));
#42993=CARTESIAN_POINT('',(38.,5.35,76.1));
#42994=CARTESIAN_POINT('',(37.9,5.35,76.));
#42995=CARTESIAN_POINT('Origin',(37.95,4.15,83.5));
#42996=CARTESIAN_POINT('',(37.9,4.1,83.5));
#42997=CARTESIAN_POINT('',(38.,4.2,77.1));
#42998=CARTESIAN_POINT('',(38.,4.2,83.5));
#42999=CARTESIAN_POINT('',(38.,4.2,77.1));
#43000=CARTESIAN_POINT('Origin',(37.95,3.3,77.05));
#43001=CARTESIAN_POINT('',(38.,-4.2,77.1));
#43002=CARTESIAN_POINT('',(38.,3.3,77.1));
#43003=CARTESIAN_POINT('',(38.,-4.2,77.1));
#43004=CARTESIAN_POINT('Origin',(37.95,-4.15,78.5));
#43005=CARTESIAN_POINT('',(38.,-4.2,78.5));
#43006=CARTESIAN_POINT('',(37.9,-4.1,78.5));
#43007=CARTESIAN_POINT('Origin',(-37.95,-4.15,78.5));
#43008=CARTESIAN_POINT('',(-38.,-4.2,77.1));
#43009=CARTESIAN_POINT('',(-38.,-4.2,78.5));
#43010=CARTESIAN_POINT('',(-38.,-4.2,77.1));
#43011=CARTESIAN_POINT('',(-37.9,-4.1,78.5));
#43012=CARTESIAN_POINT('Origin',(38.,6.6,81.));
#43013=CARTESIAN_POINT('',(38.,9.,76.5));
#43014=CARTESIAN_POINT('',(38.,9.,78.5));
#43015=CARTESIAN_POINT('',(38.,4.6,76.5));
#43016=CARTESIAN_POINT('',(38.,7.85,76.5));
#43017=CARTESIAN_POINT('',(38.,4.6,85.5));
#43018=CARTESIAN_POINT('',(38.,4.6,78.8));
#43019=CARTESIAN_POINT('',(38.,9.,85.5));
#43020=CARTESIAN_POINT('',(38.,5.65,85.5));
#43021=CARTESIAN_POINT('',(38.,9.,85.9));
#43022=CARTESIAN_POINT('',(38.,9.,83.2));
#43023=CARTESIAN_POINT('',(38.,4.2,85.9));
#43024=CARTESIAN_POINT('',(38.,7.85,85.9));
#43025=CARTESIAN_POINT('',(38.,4.2,84.9));
#43026=CARTESIAN_POINT('',(38.,4.2,83.5));
#43027=CARTESIAN_POINT('',(38.,-4.2,84.9));
#43028=CARTESIAN_POINT('',(38.,3.3,84.9));
#43029=CARTESIAN_POINT('',(38.,-4.2,85.9));
#43030=CARTESIAN_POINT('',(38.,-4.2,78.5));
#43031=CARTESIAN_POINT('',(38.,-9.,85.9));
#43032=CARTESIAN_POINT('',(38.,1.25,85.9));
#43033=CARTESIAN_POINT('',(38.,-9.,85.5));
#43034=CARTESIAN_POINT('',(38.,-9.,83.5));
#43035=CARTESIAN_POINT('',(38.,-1.25,85.5));
#43036=CARTESIAN_POINT('Origin',(-38.,9.05,76.55));
#43037=CARTESIAN_POINT('',(37.95,9.04999999999999,76.55));
#43038=CARTESIAN_POINT('',(25.6166666666671,21.3833333333336,64.2166666666671));
#43039=CARTESIAN_POINT('',(-37.9,9.,76.6));
#43040=CARTESIAN_POINT('',(-36.6583333333333,7.75833333333324,77.8416666666667));
#43041=CARTESIAN_POINT('',(37.9,9.,76.6));
#43042=CARTESIAN_POINT('',(-38.,9.,76.6));
#43043=CARTESIAN_POINT('',(25.0916666666671,-3.80833333333358,89.4083333333329));
#43044=CARTESIAN_POINT('Origin',(37.95,7.85,76.55));
#43045=CARTESIAN_POINT('',(37.9,4.7,76.6));
#43046=CARTESIAN_POINT('',(37.9,7.85,76.6));
#43047=CARTESIAN_POINT('',(38.,4.6,76.5));
#43048=CARTESIAN_POINT('',(37.825,9.17499999999999,76.675));
#43049=CARTESIAN_POINT('Origin',(-38.,9.1,76.6));
#43050=CARTESIAN_POINT('',(-37.9,4.7,76.6));
#43051=CARTESIAN_POINT('',(-37.9,1.25,76.6));
#43052=CARTESIAN_POINT('',(-38.,4.7,76.6));
#43053=CARTESIAN_POINT('Origin',(-37.95,1.25,76.55));
#43054=CARTESIAN_POINT('',(-38.,4.6,76.5));
#43055=CARTESIAN_POINT('',(-38.,1.25,76.5));
#43056=CARTESIAN_POINT('',(-38.,4.6,76.5));
#43057=CARTESIAN_POINT('Origin',(37.95,4.65,78.8));
#43058=CARTESIAN_POINT('',(37.9,4.7,85.4));
#43059=CARTESIAN_POINT('',(37.9,4.7,78.8));
#43060=CARTESIAN_POINT('',(36.675,5.92500000000003,84.175));
#43061=CARTESIAN_POINT('Origin',(37.95,-4.15,78.5));
#43062=CARTESIAN_POINT('',(37.9,-4.1,85.));
#43063=CARTESIAN_POINT('',(37.9,-4.1,85.9));
#43064=CARTESIAN_POINT('',(37.9,-4.1,78.5));
#43065=CARTESIAN_POINT('',(37.95,-4.15,85.95));
#43066=CARTESIAN_POINT('',(24.0500000000005,9.75000000000025,72.0500000000005));
#43067=CARTESIAN_POINT('',(38.2916666666666,-4.49166666666663,85.6083333333334));
#43068=CARTESIAN_POINT('',(38.,-4.2,84.9));
#43069=CARTESIAN_POINT('Origin',(37.95,3.3,84.95));
#43070=CARTESIAN_POINT('',(37.9,4.1,85.));
#43071=CARTESIAN_POINT('',(38.,4.2,84.9));
#43072=CARTESIAN_POINT('',(37.9,3.3,85.));
#43073=CARTESIAN_POINT('Origin',(37.9,4.1,85.9));
#43074=CARTESIAN_POINT('',(37.9,4.2,86.));
#43075=CARTESIAN_POINT('',(37.9,4.2,86.));
#43076=CARTESIAN_POINT('',(37.9,4.1,85.9));
#43077=CARTESIAN_POINT('',(37.9,4.1,85.9));
#43078=CARTESIAN_POINT('',(38.,4.2,85.9));
#43079=CARTESIAN_POINT('Origin',(-38.,4.15,85.95));
#43080=CARTESIAN_POINT('',(-37.95,4.15,85.95));
#43081=CARTESIAN_POINT('',(-37.9,4.1,85.9));
#43082=CARTESIAN_POINT('',(-37.55,3.74999999999999,85.55));
#43083=CARTESIAN_POINT('',(-38.,4.1,85.9));
#43084=CARTESIAN_POINT('',(-37.9,4.2,86.));
#43085=CARTESIAN_POINT('',(-38.,4.2,86.));
#43086=CARTESIAN_POINT('',(-38.4416666666667,3.6583333333333,85.4583333333333));
#43087=CARTESIAN_POINT('Origin',(37.95,4.15,83.5));
#43088=CARTESIAN_POINT('',(37.9,4.1,83.5));
#43089=CARTESIAN_POINT('Origin',(37.95,7.85,85.95));
#43090=CARTESIAN_POINT('',(37.95,9.05000000000001,85.95));
#43091=CARTESIAN_POINT('',(37.9,9.,86.));
#43092=CARTESIAN_POINT('',(25.0916666666671,-3.80833333333357,98.8083333333329));
#43093=CARTESIAN_POINT('',(37.9,7.85,86.));
#43094=CARTESIAN_POINT('',(38.6083333333333,8.39166666666664,85.2916666666667));
#43095=CARTESIAN_POINT('Origin',(36.25,0.,85.));
#43096=CARTESIAN_POINT('',(-0.875,-4.1,85.));
#43097=CARTESIAN_POINT('',(-0.875,4.1,85.));
#43098=CARTESIAN_POINT('Origin',(-38.,4.1,86.));
#43099=CARTESIAN_POINT('',(-37.9,4.1,85.));
#43100=CARTESIAN_POINT('',(-37.9,4.1,83.5));
#43101=CARTESIAN_POINT('',(-37.125,4.1,85.));
#43102=CARTESIAN_POINT('',(-37.9,4.1,83.5));
#43103=CARTESIAN_POINT('Origin',(-37.95,4.15,83.5));
#43104=CARTESIAN_POINT('',(-38.,4.2,85.9));
#43105=CARTESIAN_POINT('',(-38.,4.2,85.9));
#43106=CARTESIAN_POINT('',(-38.,4.2,84.9));
#43107=CARTESIAN_POINT('',(-38.,4.2,83.5));
#43108=CARTESIAN_POINT('',(-38.,4.2,84.9));
#43109=CARTESIAN_POINT('Origin',(-37.95,1.25,85.95));
#43110=CARTESIAN_POINT('',(-37.9,9.,86.));
#43111=CARTESIAN_POINT('',(-37.9,1.25,86.));
#43112=CARTESIAN_POINT('',(-37.95,9.05,85.95));
#43113=CARTESIAN_POINT('',(-36.6583333333333,7.75833333333324,87.2416666666667));
#43114=CARTESIAN_POINT('',(-38.,9.,85.9));
#43115=CARTESIAN_POINT('',(-39.7083333333333,7.29166666666657,84.1916666666667));
#43116=CARTESIAN_POINT('',(-38.,1.25,85.9));
#43117=CARTESIAN_POINT('Origin',(-38.,9.1,86.));
#43118=CARTESIAN_POINT('',(-38.,9.,86.));
#43119=CARTESIAN_POINT('',(-6.,6.1,86.));
#43120=CARTESIAN_POINT('',(6.,6.1,86.));
#43121=CARTESIAN_POINT('',(-16.,6.1,86.));
#43122=CARTESIAN_POINT('',(-6.,7.7,86.));
#43123=CARTESIAN_POINT('Origin',(-6.,6.9,86.));
#43124=CARTESIAN_POINT('',(6.,7.7,86.));
#43125=CARTESIAN_POINT('',(-22.,7.7,86.));
#43126=CARTESIAN_POINT('Origin',(6.,6.9,86.));
#43127=CARTESIAN_POINT('Origin',(-38.,9.05,85.95));
#43128=CARTESIAN_POINT('',(37.9,9.1,85.9));
#43129=CARTESIAN_POINT('',(24.8333333333338,22.1666666666669,72.8333333333338));
#43130=CARTESIAN_POINT('',(-37.9,9.1,85.9));
#43131=CARTESIAN_POINT('',(-38.,9.1,85.9));
#43132=CARTESIAN_POINT('',(-37.5,9.50000000000001,85.5));
#43133=CARTESIAN_POINT('Origin',(-37.95,9.05,83.2));
#43134=CARTESIAN_POINT('',(-37.9,9.1,85.5));
#43135=CARTESIAN_POINT('',(-37.9,9.1,83.2));
#43136=CARTESIAN_POINT('',(-37.95,9.05,85.45));
#43137=CARTESIAN_POINT('',(-38.3333333333333,8.66666666666666,85.0666666666667));
#43138=CARTESIAN_POINT('',(-38.,9.,85.5));
#43139=CARTESIAN_POINT('',(-39.2416666666667,7.75833333333322,86.7416666666667));
#43140=CARTESIAN_POINT('',(-38.,9.,83.2));
#43141=CARTESIAN_POINT('Origin',(-38.,9.05,85.45));
#43142=CARTESIAN_POINT('',(37.95,9.05,85.45));
#43143=CARTESIAN_POINT('',(37.9,9.,85.4));
#43144=CARTESIAN_POINT('',(24.7250000000004,-4.17500000000027,72.2250000000004));
#43145=CARTESIAN_POINT('',(-37.9,9.,85.4));
#43146=CARTESIAN_POINT('',(-38.,9.,85.4));
#43147=CARTESIAN_POINT('',(-36.2916666666666,7.39166666666655,83.7916666666666));
#43148=CARTESIAN_POINT('',(37.9,9.1,85.5));
#43149=CARTESIAN_POINT('',(-38.,9.1,85.5));
#43150=CARTESIAN_POINT('',(25.6666666666671,21.3333333333336,97.7333333333329));
#43151=CARTESIAN_POINT('Origin',(-37.95,-0.95,85.45));
#43152=CARTESIAN_POINT('',(-37.9,4.7,85.4));
#43153=CARTESIAN_POINT('',(-37.9,-0.95,85.4));
#43154=CARTESIAN_POINT('',(-38.,4.6,85.5));
#43155=CARTESIAN_POINT('',(-38.,4.6,85.5));
#43156=CARTESIAN_POINT('',(-38.,-0.95,85.5));
#43157=CARTESIAN_POINT('Origin',(-38.,4.7,85.4));
#43158=CARTESIAN_POINT('',(37.9,5.65,85.4));
#43159=CARTESIAN_POINT('',(-38.,4.7,85.4));
#43160=CARTESIAN_POINT('',(6.,6.1,85.4));
#43161=CARTESIAN_POINT('',(-6.,6.1,85.4));
#43162=CARTESIAN_POINT('',(-16.,6.1,85.4));
#43163=CARTESIAN_POINT('',(6.,7.7,85.4));
#43164=CARTESIAN_POINT('Origin',(6.,6.9,85.4));
#43165=CARTESIAN_POINT('',(-6.,7.7,85.4));
#43166=CARTESIAN_POINT('',(-22.,7.7,85.4));
#43167=CARTESIAN_POINT('Origin',(-6.,6.9,85.4));
#43168=CARTESIAN_POINT('Origin',(37.95,5.65,85.45));
#43169=CARTESIAN_POINT('',(38.1416666666667,8.8583333333333,85.6416666666667));
#43170=CARTESIAN_POINT('Origin',(37.95,9.05,83.2));
#43171=CARTESIAN_POINT('',(37.9,9.1,83.2));
#43172=CARTESIAN_POINT('Origin',(-37.95,-3.3,77.05));
#43173=CARTESIAN_POINT('',(-38.,4.2,77.1));
#43174=CARTESIAN_POINT('',(-38.,-3.3,77.1));
#43175=CARTESIAN_POINT('',(-38.,4.2,77.1));
#43176=CARTESIAN_POINT('Origin',(-37.95,4.15,83.5));
#43177=CARTESIAN_POINT('',(-38.,4.2,83.5));
#43178=CARTESIAN_POINT('Origin',(-38.,-6.6,81.));
#43179=CARTESIAN_POINT('',(-38.,-4.6,76.5));
#43180=CARTESIAN_POINT('',(-38.,-5.65,76.5));
#43181=CARTESIAN_POINT('',(-38.,-4.6,85.5));
#43182=CARTESIAN_POINT('',(-38.,-4.6,83.2));
#43183=CARTESIAN_POINT('',(-38.,-9.,85.5));
#43184=CARTESIAN_POINT('',(-38.,-7.85,85.5));
#43185=CARTESIAN_POINT('',(-38.,-9.,85.9));
#43186=CARTESIAN_POINT('',(-38.,-9.,83.5));
#43187=CARTESIAN_POINT('',(-38.,-4.2,85.9));
#43188=CARTESIAN_POINT('',(-38.,-5.35,85.9));
#43189=CARTESIAN_POINT('',(-38.,-4.2,84.9));
#43190=CARTESIAN_POINT('',(-38.,-4.2,78.5));
#43191=CARTESIAN_POINT('',(-38.,-3.3,84.9));
#43192=CARTESIAN_POINT('',(-38.,4.6,78.8));
#43193=CARTESIAN_POINT('Origin',(-37.95,4.65,78.8));
#43194=CARTESIAN_POINT('',(-37.9,4.7,78.8));
#43195=CARTESIAN_POINT('Origin',(-38.,4.7,76.6));
#43196=CARTESIAN_POINT('Origin',(-38.,-4.2,85.9));
#43197=CARTESIAN_POINT('',(-37.9,-4.1,85.9));
#43198=CARTESIAN_POINT('',(-37.9,-4.2,86.));
#43199=CARTESIAN_POINT('',(-37.9,-4.1,85.9));
#43200=CARTESIAN_POINT('',(-38.,-4.2,85.9));
#43201=CARTESIAN_POINT('',(-37.9,-4.2,86.));
#43202=CARTESIAN_POINT('Origin',(-37.95,-4.15,78.5));
#43203=CARTESIAN_POINT('',(-37.9,-4.1,85.));
#43204=CARTESIAN_POINT('',(-37.9,-4.1,78.5));
#43205=CARTESIAN_POINT('',(-37.9,-4.1,85.));
#43206=CARTESIAN_POINT('Origin',(-37.95,-5.35,85.95));
#43207=CARTESIAN_POINT('',(-37.95,-9.05,85.95));
#43208=CARTESIAN_POINT('',(-37.9,-9.,86.));
#43209=CARTESIAN_POINT('',(-37.3416666666666,-8.44166666666665,86.5583333333333));
#43210=CARTESIAN_POINT('',(-37.9,-5.35,86.));
#43211=CARTESIAN_POINT('',(-38.975,-8.025,84.925));
#43212=CARTESIAN_POINT('Origin',(-38.,-4.15,85.95));
#43213=CARTESIAN_POINT('',(-38.,-4.1,85.9));
#43214=CARTESIAN_POINT('',(37.9,-4.2,86.));
#43215=CARTESIAN_POINT('',(-38.,-4.2,86.));
#43216=CARTESIAN_POINT('',(37.9,-4.2,86.));
#43217=CARTESIAN_POINT('Origin',(-37.95,-3.3,84.95));
#43218=CARTESIAN_POINT('',(-37.9,-3.3,85.));
#43219=CARTESIAN_POINT('Origin',(37.95,1.25,85.95));
#43220=CARTESIAN_POINT('',(37.9,-9.,86.));
#43221=CARTESIAN_POINT('',(37.9,1.25,86.));
#43222=CARTESIAN_POINT('',(37.95,-9.05,85.95));
#43223=CARTESIAN_POINT('',(23.5750000000004,5.32500000000035,100.325));
#43224=CARTESIAN_POINT('',(40.075,-6.92499999999987,83.825));
#43225=CARTESIAN_POINT('Origin',(-36.25,0.,85.));
#43226=CARTESIAN_POINT('',(-37.125,-4.1,85.));
#43227=CARTESIAN_POINT('Origin',(-38.,-4.1,76.));
#43228=CARTESIAN_POINT('Origin',(37.95,-9.05,83.5));
#43229=CARTESIAN_POINT('',(37.9,-9.1,85.9));
#43230=CARTESIAN_POINT('',(24.8833333333338,-22.1166666666669,72.8833333333338));
#43231=CARTESIAN_POINT('',(37.9,-9.1,85.5));
#43232=CARTESIAN_POINT('',(37.9,-9.1,83.5));
#43233=CARTESIAN_POINT('',(37.95,-9.05,85.45));
#43234=CARTESIAN_POINT('',(25.6166666666671,-21.3833333333336,97.7833333333329));
#43235=CARTESIAN_POINT('',(38.925,-8.07499999999991,86.425));
#43236=CARTESIAN_POINT('Origin',(-37.95,-4.65,83.2));
#43237=CARTESIAN_POINT('',(-37.0416666666667,-5.55833333333334,84.5416666666667));
#43238=CARTESIAN_POINT('',(-38.,-4.6,76.5));
#43239=CARTESIAN_POINT('Origin',(-37.95,-5.65,76.55));
#43240=CARTESIAN_POINT('Origin',(37.95,-1.25,85.45));
#43241=CARTESIAN_POINT('',(37.9,-9.,85.4));
#43242=CARTESIAN_POINT('',(23.9916666666671,4.90833333333365,71.4916666666671));
#43243=CARTESIAN_POINT('',(37.9,-1.25,85.4));
#43244=CARTESIAN_POINT('Origin',(-38.,-9.1,85.4));
#43245=CARTESIAN_POINT('',(-37.9,-9.,85.4));
#43246=CARTESIAN_POINT('',(-38.,-9.,85.4));
#43247=CARTESIAN_POINT('',(-37.9,-7.85,85.4));
#43248=CARTESIAN_POINT('',(6.,-7.7,85.4));
#43249=CARTESIAN_POINT('',(-6.,-7.7,85.4));
#43250=CARTESIAN_POINT('',(-16.,-7.7,85.4));
#43251=CARTESIAN_POINT('',(6.,-6.1,85.4));
#43252=CARTESIAN_POINT('Origin',(6.,-6.9,85.4));
#43253=CARTESIAN_POINT('',(-6.,-6.1,85.4));
#43254=CARTESIAN_POINT('',(-22.,-6.1,85.4));
#43255=CARTESIAN_POINT('Origin',(-6.,-6.9,85.4));
#43256=CARTESIAN_POINT('Origin',(-38.,-9.05,85.45));
#43257=CARTESIAN_POINT('',(-37.9,-9.1,85.5));
#43258=CARTESIAN_POINT('',(-38.,-9.1,85.5));
#43259=CARTESIAN_POINT('',(-37.95,-9.05,85.45));
#43260=CARTESIAN_POINT('',(-38.2833333333333,-8.71666666666668,85.1166666666667));
#43261=CARTESIAN_POINT('',(-37.7583333333333,-8.85833333333333,85.2583333333333));
#43262=CARTESIAN_POINT('Origin',(-37.95,-7.85,85.45));
#43263=CARTESIAN_POINT('',(-37.825,-9.17499999999998,85.325));
#43264=CARTESIAN_POINT('Origin',(-37.95,-9.05,83.5));
#43265=CARTESIAN_POINT('',(-37.9,-9.1,85.9));
#43266=CARTESIAN_POINT('',(-37.9,-9.1,83.5));
#43267=CARTESIAN_POINT('',(-37.55,-9.44999999999999,85.55));
#43268=CARTESIAN_POINT('Origin',(-38.,-9.05,85.95));
#43269=CARTESIAN_POINT('',(-38.,-9.1,85.9));
#43270=CARTESIAN_POINT('',(-38.,-9.,86.));
#43271=CARTESIAN_POINT('Origin',(-38.,-4.1,86.));
#43272=CARTESIAN_POINT('',(-6.,-7.7,86.));
#43273=CARTESIAN_POINT('',(6.,-7.7,86.));
#43274=CARTESIAN_POINT('',(-16.,-7.7,86.));
#43275=CARTESIAN_POINT('',(-6.,-6.1,86.));
#43276=CARTESIAN_POINT('Origin',(-6.,-6.9,86.));
#43277=CARTESIAN_POINT('',(6.,-6.1,86.));
#43278=CARTESIAN_POINT('',(-22.,-6.1,86.));
#43279=CARTESIAN_POINT('Origin',(6.,-6.9,86.));
#43280=CARTESIAN_POINT('Origin',(-16.,6.15,85.45));
#43281=CARTESIAN_POINT('',(6.,6.2,85.5));
#43282=CARTESIAN_POINT('',(6.,6.2,85.5));
#43283=CARTESIAN_POINT('',(-6.,6.2,85.5));
#43284=CARTESIAN_POINT('',(-6.,6.1,85.4));
#43285=CARTESIAN_POINT('',(-16.,6.2,85.5));
#43286=CARTESIAN_POINT('Origin',(6.,6.9,85.45));
#43287=CARTESIAN_POINT('',(6.,7.6,85.5));
#43288=CARTESIAN_POINT('',(6.,7.6,85.5));
#43289=CARTESIAN_POINT('Origin',(6.,6.9,85.5));
#43290=CARTESIAN_POINT('Origin',(-22.,7.65,85.45));
#43291=CARTESIAN_POINT('',(-6.,7.6,85.5));
#43292=CARTESIAN_POINT('',(-6.,7.6,85.5));
#43293=CARTESIAN_POINT('',(-22.,7.6,85.5));
#43294=CARTESIAN_POINT('Origin',(-6.,6.9,85.45));
#43295=CARTESIAN_POINT('Origin',(-6.,6.9,85.5));
#43296=CARTESIAN_POINT('Origin',(6.,6.9,86.));
#43297=CARTESIAN_POINT('',(6.,6.2,85.9));
#43298=CARTESIAN_POINT('',(6.,6.2,86.));
#43299=CARTESIAN_POINT('',(6.,7.6,85.9));
#43300=CARTESIAN_POINT('Origin',(6.,6.9,85.9));
#43301=CARTESIAN_POINT('',(6.,7.6,86.));
#43302=CARTESIAN_POINT('Origin',(6.,6.2,86.));
#43303=CARTESIAN_POINT('',(-6.,6.2,85.9));
#43304=CARTESIAN_POINT('',(-6.,6.2,86.));
#43305=CARTESIAN_POINT('',(-16.,6.2,85.9));
#43306=CARTESIAN_POINT('Origin',(-16.,6.15,85.95));
#43307=CARTESIAN_POINT('',(-6.,6.2,85.9));
#43308=CARTESIAN_POINT('',(6.,6.1,86.));
#43309=CARTESIAN_POINT('Origin',(-6.,6.9,85.95));
#43310=CARTESIAN_POINT('',(-6.,7.6,85.9));
#43311=CARTESIAN_POINT('',(-6.,7.6,85.9));
#43312=CARTESIAN_POINT('Origin',(-6.,6.9,85.9));
#43313=CARTESIAN_POINT('Origin',(-22.,7.65,85.95));
#43314=CARTESIAN_POINT('',(6.,7.6,85.9));
#43315=CARTESIAN_POINT('',(-22.,7.6,85.9));
#43316=CARTESIAN_POINT('Origin',(6.,6.9,85.95));
#43317=CARTESIAN_POINT('Origin',(-6.,6.9,86.));
#43318=CARTESIAN_POINT('',(-6.,7.6,86.));
#43319=CARTESIAN_POINT('Origin',(-16.,-7.65,85.45));
#43320=CARTESIAN_POINT('',(6.,-7.6,85.5));
#43321=CARTESIAN_POINT('',(6.,-7.6,85.5));
#43322=CARTESIAN_POINT('',(-6.,-7.6,85.5));
#43323=CARTESIAN_POINT('',(-6.,-7.7,85.4));
#43324=CARTESIAN_POINT('',(-16.,-7.6,85.5));
#43325=CARTESIAN_POINT('Origin',(6.,-6.9,85.45));
#43326=CARTESIAN_POINT('',(6.,-6.2,85.5));
#43327=CARTESIAN_POINT('',(6.,-6.2,85.5));
#43328=CARTESIAN_POINT('Origin',(6.,-6.9,85.5));
#43329=CARTESIAN_POINT('Origin',(-22.,-6.15,85.45));
#43330=CARTESIAN_POINT('',(-6.,-6.2,85.5));
#43331=CARTESIAN_POINT('',(-6.,-6.2,85.5));
#43332=CARTESIAN_POINT('',(-22.,-6.2,85.5));
#43333=CARTESIAN_POINT('Origin',(-6.,-6.9,85.45));
#43334=CARTESIAN_POINT('Origin',(-6.,-6.9,85.5));
#43335=CARTESIAN_POINT('Origin',(6.,-6.9,86.));
#43336=CARTESIAN_POINT('',(6.,-7.6,85.9));
#43337=CARTESIAN_POINT('',(6.,-7.6,86.));
#43338=CARTESIAN_POINT('',(6.,-6.2,85.9));
#43339=CARTESIAN_POINT('Origin',(6.,-6.9,85.9));
#43340=CARTESIAN_POINT('',(6.,-6.2,86.));
#43341=CARTESIAN_POINT('Origin',(6.,-7.6,86.));
#43342=CARTESIAN_POINT('',(-6.,-7.6,85.9));
#43343=CARTESIAN_POINT('',(-6.,-7.6,86.));
#43344=CARTESIAN_POINT('',(-16.,-7.6,85.9));
#43345=CARTESIAN_POINT('Origin',(-16.,-7.65,85.95));
#43346=CARTESIAN_POINT('',(-6.,-7.6,85.9));
#43347=CARTESIAN_POINT('',(6.,-7.7,86.));
#43348=CARTESIAN_POINT('Origin',(-6.,-6.9,85.95));
#43349=CARTESIAN_POINT('',(-6.,-6.2,85.9));
#43350=CARTESIAN_POINT('',(-6.,-6.2,85.9));
#43351=CARTESIAN_POINT('Origin',(-6.,-6.9,85.9));
#43352=CARTESIAN_POINT('Origin',(-22.,-6.15,85.95));
#43353=CARTESIAN_POINT('',(6.,-6.2,85.9));
#43354=CARTESIAN_POINT('',(-22.,-6.2,85.9));
#43355=CARTESIAN_POINT('Origin',(6.,-6.9,85.95));
#43356=CARTESIAN_POINT('Origin',(-6.,-6.9,86.));
#43357=CARTESIAN_POINT('',(-6.,-6.2,86.));
#43358=CARTESIAN_POINT('Origin',(-6.,-6.2,86.));
#43359=CARTESIAN_POINT('Origin',(-6.,7.6,86.));
#43360=CARTESIAN_POINT('Origin',(-38.,-9.1,86.));
#43361=CARTESIAN_POINT('Origin',(37.95,9.05,78.5));
#43362=CARTESIAN_POINT('Origin',(-38.,9.1,85.4));
#43363=CARTESIAN_POINT('Origin',(-38.,4.1,76.));
#71454=UNCERTAINTY_MEASURE_WITH_UNIT(LENGTH_MEASURE(0.001),#71493,
'DISTANCE_ACCURACY_VALUE',
'Maximum model space distance between geometric entities at asserted c
onnectivities');
#71471=UNCERTAINTY_MEASURE_WITH_UNIT(LENGTH_MEASURE(0.001),#71493,
'DISTANCE_ACCURACY_VALUE',
'Maximum model space distance between geometric entities at asserted c
onnectivities');
#71475=(
GEOMETRIC_REPRESENTATION_CONTEXT(3)
GLOBAL_UNCERTAINTY_ASSIGNED_CONTEXT((#71454))
GLOBAL_UNIT_ASSIGNED_CONTEXT((#71493,#71495,#71496))
REPRESENTATION_CONTEXT('','3D')
);
#71492=(
GEOMETRIC_REPRESENTATION_CONTEXT(3)
GLOBAL_UNCERTAINTY_ASSIGNED_CONTEXT((#71471))
GLOBAL_UNIT_ASSIGNED_CONTEXT((#71493,#71495,#71496))
REPRESENTATION_CONTEXT('','3D')
);
#71493=(
LENGTH_UNIT()
NAMED_UNIT(*)
SI_UNIT(.CENTI.,.METRE.)
);
#71495=(
NAMED_UNIT(*)
PLANE_ANGLE_UNIT()
SI_UNIT($,.RADIAN.)
);
#71496=(
NAMED_UNIT(*)
SI_UNIT($,.STERADIAN.)
SOLID_ANGLE_UNIT()
);
#71500=SHAPE_DEFINITION_REPRESENTATION(#71520,#71605);
#71520=PRODUCT_DEFINITION_SHAPE('',$,#71626);
#71605=SHAPE_REPRESENTATION('',(#29181),#71475);
#71622=PRODUCT_DEFINITION_CONTEXT('part definition',#71684,'design');
#71626=PRODUCT_DEFINITION('2026-10-19-03-21-51-757',
'04_Height-Adjustable_Bed_Twin_C100x50x6',#71646,#71622);
#71646=PRODUCT_DEFINITION_FORMATION('',$,#71689);
#71684=APPLICATION_CONTEXT(
'Core Data for Automotive Mechanical Design Process');
#71685=PRODUCT_CONTEXT('part definition',#71684,'mechanical');
#71689=PRODUCT('2026-10-19-03-21-51-757',
'04_Height-Adjustable_Bed_Twin_C100x50x6',$,(#71685));
#71895=COLOUR_RGB('Off White',0.89,0.88,0.83);
#71896=FILL_AREA_STYLE_COLOUR('',#71895);
#71897=FILL_AREA_STYLE('',(#71896));
#71898=SURFACE_STYLE_FILL_AREA(#71897);
#71899=SURFACE_SIDE_STYLE('',(#71898));
#71900=SURFACE_STYLE_USAGE(.BOTH.,#71899);
#71901=PRESENTATION_STYLE_ASSIGNMENT((#71900));
ENDSEC;
END-ISO-10303-21;
